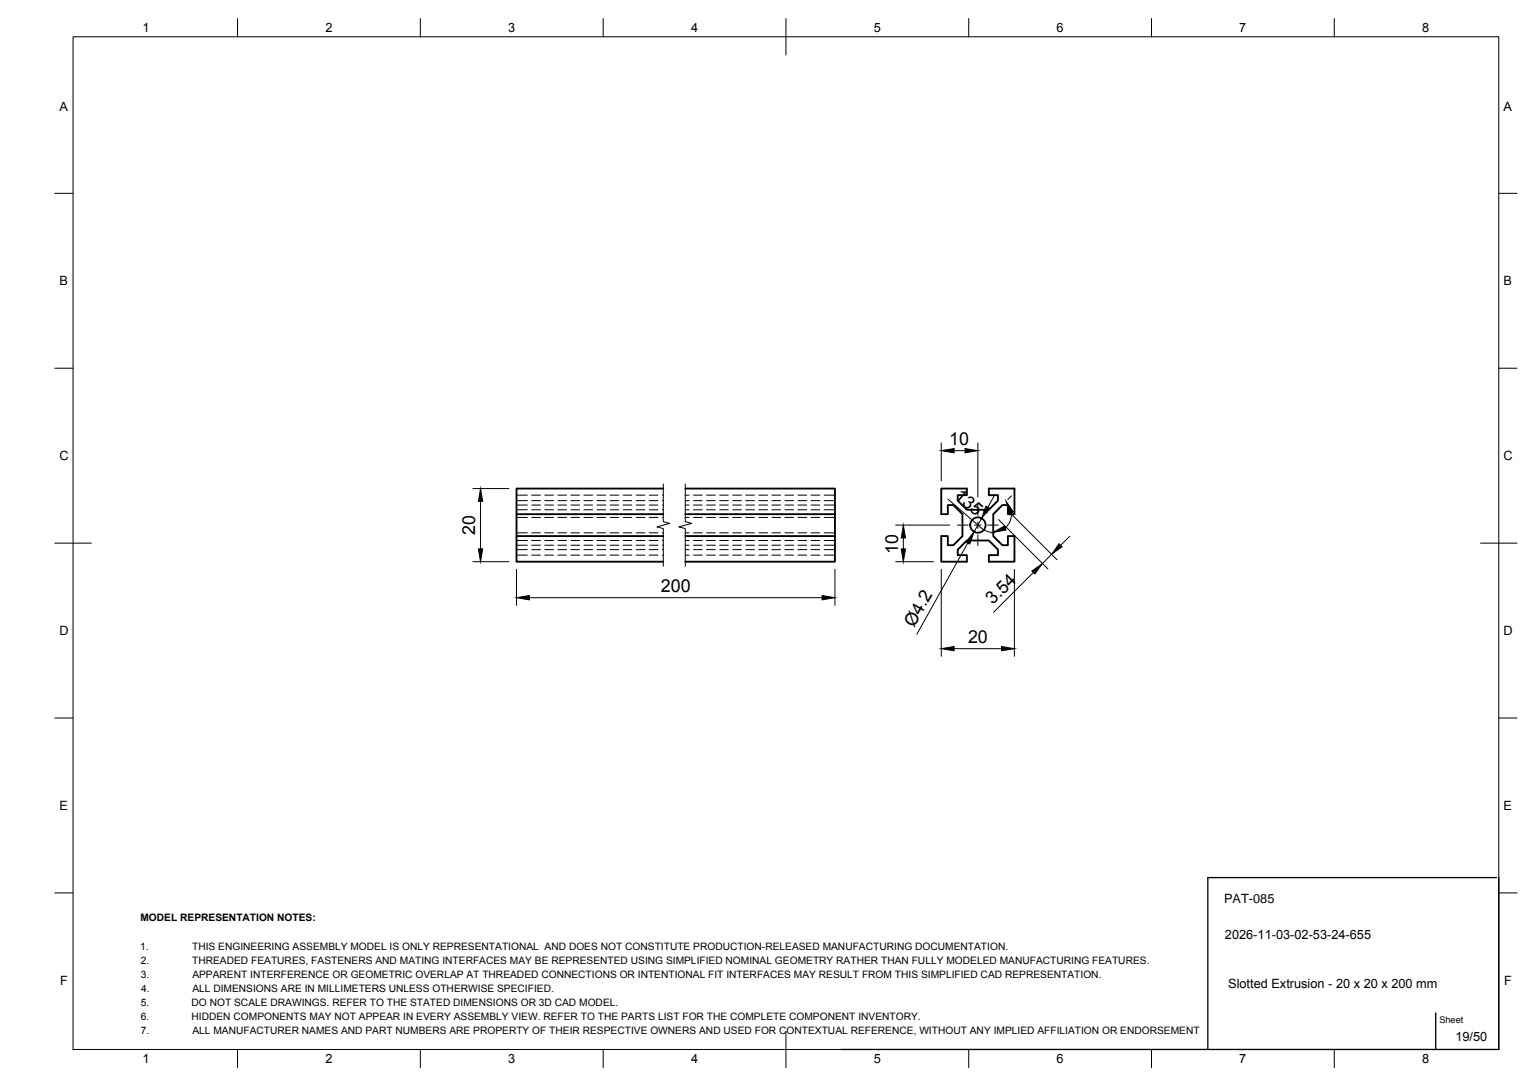
ISO-10303-21;
HEADER;
/* Generated by software containing ST-Developer
 * from STEP Tools, Inc. (www.steptools.com) 
 */

FILE_DESCRIPTION(
/* description */ ('Rack and pinion manual slide'),
/* implementation_level */ '2;1');

FILE_NAME(
/* name */ 'Slotted Extrusion - 20 x 20 x 200 mm.step',
/* time_stamp */ '2026-10-28T03:22:49-07:00',
/* author */ (''),
/* organization */ (''),
/* preprocessor_version */ 'ST-DEVELOPER v20.2',
/* originating_system */ 'Autodesk Translation Framework v15.17.0.0',
/* authorisation */ '');

FILE_SCHEMA (('AUTOMOTIVE_DESIGN { 1 0 10303 214 3 1 1 }'));
ENDSEC;

DATA;
#10=MECHANICAL_DESIGN_GEOMETRIC_PRESENTATION_REPRESENTATION('',(#746),#34851);
#654=SHAPE_REPRESENTATION_RELATIONSHIP('SRR','None',#35089,#700);
#700=ADVANCED_BREP_SHAPE_REPRESENTATION('',(#799),#34814);
#746=STYLED_ITEM('',(#35425),#799);
#799=MANIFOLD_SOLID_BREP('Body1',#13766);
#957=FACE_BOUND('',#2598,.T.);
#958=FACE_BOUND('',#2600,.T.);
#1128=PLANE('',#14628);
#1129=PLANE('',#14629);
#1130=PLANE('',#14630);
#1131=PLANE('',#14631);
#1132=PLANE('',#14632);
#1133=PLANE('',#14633);
#1134=PLANE('',#14634);
#1135=PLANE('',#14635);
#1136=PLANE('',#14636);
#1137=PLANE('',#14637);
#1138=PLANE('',#14638);
#1139=PLANE('',#14639);
#1140=PLANE('',#14640);
#1141=PLANE('',#14641);
#1142=PLANE('',#14642);
#1143=PLANE('',#14643);
#1144=PLANE('',#14644);
#1145=PLANE('',#14645);
#1146=PLANE('',#14646);
#1147=PLANE('',#14647);
#1148=PLANE('',#14648);
#1149=PLANE('',#14649);
#1150=PLANE('',#14650);
#1151=PLANE('',#14651);
#1152=PLANE('',#14652);
#1153=PLANE('',#14653);
#1154=PLANE('',#14654);
#1155=PLANE('',#14655);
#1156=PLANE('',#14656);
#1157=PLANE('',#14657);
#1158=PLANE('',#14658);
#1159=PLANE('',#14659);
#1160=PLANE('',#14660);
#1161=PLANE('',#14661);
#1162=PLANE('',#14662);
#1163=PLANE('',#14663);
#1164=PLANE('',#14667);
#1165=PLANE('',#14668);
#1166=PLANE('',#14669);
#1167=PLANE('',#14670);
#1168=PLANE('',#14671);
#1169=PLANE('',#14672);
#1170=PLANE('',#14673);
#1171=PLANE('',#14674);
#1172=PLANE('',#14675);
#1173=PLANE('',#14676);
#1689=FACE_OUTER_BOUND('',#2552,.T.);
#1690=FACE_OUTER_BOUND('',#2553,.T.);
#1691=FACE_OUTER_BOUND('',#2554,.T.);
#1692=FACE_OUTER_BOUND('',#2555,.T.);
#1693=FACE_OUTER_BOUND('',#2556,.T.);
#1694=FACE_OUTER_BOUND('',#2557,.T.);
#1695=FACE_OUTER_BOUND('',#2558,.T.);
#1696=FACE_OUTER_BOUND('',#2559,.T.);
#1697=FACE_OUTER_BOUND('',#2560,.T.);
#1698=FACE_OUTER_BOUND('',#2561,.T.);
#1699=FACE_OUTER_BOUND('',#2562,.T.);
#1700=FACE_OUTER_BOUND('',#2563,.T.);
#1701=FACE_OUTER_BOUND('',#2564,.T.);
#1702=FACE_OUTER_BOUND('',#2565,.T.);
#1703=FACE_OUTER_BOUND('',#2566,.T.);
#1704=FACE_OUTER_BOUND('',#2567,.T.);
#1705=FACE_OUTER_BOUND('',#2568,.T.);
#1706=FACE_OUTER_BOUND('',#2569,.T.);
#1707=FACE_OUTER_BOUND('',#2570,.T.);
#1708=FACE_OUTER_BOUND('',#2571,.T.);
#1709=FACE_OUTER_BOUND('',#2572,.T.);
#1710=FACE_OUTER_BOUND('',#2573,.T.);
#1711=FACE_OUTER_BOUND('',#2574,.T.);
#1712=FACE_OUTER_BOUND('',#2575,.T.);
#1713=FACE_OUTER_BOUND('',#2576,.T.);
#1714=FACE_OUTER_BOUND('',#2577,.T.);
#1715=FACE_OUTER_BOUND('',#2578,.T.);
#1716=FACE_OUTER_BOUND('',#2579,.T.);
#1717=FACE_OUTER_BOUND('',#2580,.T.);
#1718=FACE_OUTER_BOUND('',#2581,.T.);
#1719=FACE_OUTER_BOUND('',#2582,.T.);
#1720=FACE_OUTER_BOUND('',#2583,.T.);
#1721=FACE_OUTER_BOUND('',#2584,.T.);
#1722=FACE_OUTER_BOUND('',#2585,.T.);
#1723=FACE_OUTER_BOUND('',#2586,.T.);
#1724=FACE_OUTER_BOUND('',#2587,.T.);
#1725=FACE_OUTER_BOUND('',#2588,.T.);
#1726=FACE_OUTER_BOUND('',#2589,.T.);
#1727=FACE_OUTER_BOUND('',#2590,.T.);
#1728=FACE_OUTER_BOUND('',#2591,.T.);
#1729=FACE_OUTER_BOUND('',#2592,.T.);
#1730=FACE_OUTER_BOUND('',#2593,.T.);
#1731=FACE_OUTER_BOUND('',#2594,.T.);
#1732=FACE_OUTER_BOUND('',#2595,.T.);
#1733=FACE_OUTER_BOUND('',#2596,.T.);
#1734=FACE_OUTER_BOUND('',#2597,.T.);
#1735=FACE_OUTER_BOUND('',#2599,.T.);
#2552=EDGE_LOOP('',(#9942,#9943,#9944,#9945));
#2553=EDGE_LOOP('',(#9946,#9947,#9948,#9949));
#2554=EDGE_LOOP('',(#9950,#9951,#9952,#9953));
#2555=EDGE_LOOP('',(#9954,#9955,#9956,#9957));
#2556=EDGE_LOOP('',(#9958,#9959,#9960,#9961));
#2557=EDGE_LOOP('',(#9962,#9963,#9964,#9965));
#2558=EDGE_LOOP('',(#9966,#9967,#9968,#9969));
#2559=EDGE_LOOP('',(#9970,#9971,#9972,#9973));
#2560=EDGE_LOOP('',(#9974,#9975,#9976,#9977));
#2561=EDGE_LOOP('',(#9978,#9979,#9980,#9981));
#2562=EDGE_LOOP('',(#9982,#9983,#9984,#9985));
#2563=EDGE_LOOP('',(#9986,#9987,#9988,#9989));
#2564=EDGE_LOOP('',(#9990,#9991,#9992,#9993));
#2565=EDGE_LOOP('',(#9994,#9995,#9996,#9997));
#2566=EDGE_LOOP('',(#9998,#9999,#10000,#10001));
#2567=EDGE_LOOP('',(#10002,#10003,#10004,#10005));
#2568=EDGE_LOOP('',(#10006,#10007,#10008,#10009));
#2569=EDGE_LOOP('',(#10010,#10011,#10012,#10013));
#2570=EDGE_LOOP('',(#10014,#10015,#10016,#10017));
#2571=EDGE_LOOP('',(#10018,#10019,#10020,#10021));
#2572=EDGE_LOOP('',(#10022,#10023,#10024,#10025));
#2573=EDGE_LOOP('',(#10026,#10027,#10028,#10029));
#2574=EDGE_LOOP('',(#10030,#10031,#10032,#10033));
#2575=EDGE_LOOP('',(#10034,#10035,#10036,#10037));
#2576=EDGE_LOOP('',(#10038,#10039,#10040,#10041));
#2577=EDGE_LOOP('',(#10042,#10043,#10044,#10045));
#2578=EDGE_LOOP('',(#10046,#10047,#10048,#10049));
#2579=EDGE_LOOP('',(#10050,#10051,#10052,#10053));
#2580=EDGE_LOOP('',(#10054,#10055,#10056,#10057));
#2581=EDGE_LOOP('',(#10058,#10059,#10060,#10061));
#2582=EDGE_LOOP('',(#10062,#10063,#10064,#10065));
#2583=EDGE_LOOP('',(#10066,#10067,#10068,#10069));
#2584=EDGE_LOOP('',(#10070,#10071,#10072,#10073));
#2585=EDGE_LOOP('',(#10074,#10075,#10076,#10077));
#2586=EDGE_LOOP('',(#10078,#10079,#10080,#10081));
#2587=EDGE_LOOP('',(#10082,#10083,#10084,#10085));
#2588=EDGE_LOOP('',(#10086,#10087,#10088,#10089));
#2589=EDGE_LOOP('',(#10090,#10091,#10092,#10093));
#2590=EDGE_LOOP('',(#10094,#10095,#10096,#10097));
#2591=EDGE_LOOP('',(#10098,#10099,#10100,#10101));
#2592=EDGE_LOOP('',(#10102,#10103,#10104,#10105));
#2593=EDGE_LOOP('',(#10106,#10107,#10108,#10109));
#2594=EDGE_LOOP('',(#10110,#10111,#10112,#10113));
#2595=EDGE_LOOP('',(#10114,#10115,#10116,#10117));
#2596=EDGE_LOOP('',(#10118,#10119,#10120,#10121));
#2597=EDGE_LOOP('',(#10122,#10123,#10124,#10125,#10126,#10127,#10128,#10129,
#10130,#10131,#10132,#10133,#10134,#10135,#10136,#10137,#10138,#10139,#10140,
#10141,#10142,#10143,#10144,#10145,#10146,#10147,#10148,#10149,#10150,#10151,
#10152,#10153,#10154,#10155,#10156,#10157,#10158,#10159,#10160,#10161,#10162,
#10163,#10164,#10165));
#2598=EDGE_LOOP('',(#10166));
#2599=EDGE_LOOP('',(#10167,#10168,#10169,#10170,#10171,#10172,#10173,#10174,
#10175,#10176,#10177,#10178,#10179,#10180,#10181,#10182,#10183,#10184,#10185,
#10186,#10187,#10188,#10189,#10190,#10191,#10192,#10193,#10194,#10195,#10196,
#10197,#10198,#10199,#10200,#10201,#10202,#10203,#10204,#10205,#10206,#10207,
#10208,#10209,#10210));
#2600=EDGE_LOOP('',(#10211));
#3438=LINE('',#20221,#4729);
#3439=LINE('',#20223,#4730);
#3440=LINE('',#20225,#4731);
#3441=LINE('',#20226,#4732);
#3442=LINE('',#20229,#4733);
#3443=LINE('',#20231,#4734);
#3444=LINE('',#20232,#4735);
#3445=LINE('',#20235,#4736);
#3446=LINE('',#20237,#4737);
#3447=LINE('',#20238,#4738);
#3448=LINE('',#20241,#4739);
#3449=LINE('',#20243,#4740);
#3450=LINE('',#20244,#4741);
#3451=LINE('',#20247,#4742);
#3452=LINE('',#20249,#4743);
#3453=LINE('',#20250,#4744);
#3454=LINE('',#20253,#4745);
#3455=LINE('',#20255,#4746);
#3456=LINE('',#20256,#4747);
#3457=LINE('',#20259,#4748);
#3458=LINE('',#20261,#4749);
#3459=LINE('',#20262,#4750);
#3460=LINE('',#20265,#4751);
#3461=LINE('',#20267,#4752);
#3462=LINE('',#20268,#4753);
#3463=LINE('',#20271,#4754);
#3464=LINE('',#20273,#4755);
#3465=LINE('',#20274,#4756);
#3466=LINE('',#20278,#4757);
#3467=LINE('',#20280,#4758);
#3468=LINE('',#20282,#4759);
#3469=LINE('',#20283,#4760);
#3470=LINE('',#20286,#4761);
#3471=LINE('',#20288,#4762);
#3472=LINE('',#20289,#4763);
#3473=LINE('',#20292,#4764);
#3474=LINE('',#20294,#4765);
#3475=LINE('',#20295,#4766);
#3476=LINE('',#20298,#4767);
#3477=LINE('',#20300,#4768);
#3478=LINE('',#20301,#4769);
#3479=LINE('',#20304,#4770);
#3480=LINE('',#20306,#4771);
#3481=LINE('',#20307,#4772);
#3482=LINE('',#20310,#4773);
#3483=LINE('',#20312,#4774);
#3484=LINE('',#20313,#4775);
#3485=LINE('',#20316,#4776);
#3486=LINE('',#20318,#4777);
#3487=LINE('',#20319,#4778);
#3488=LINE('',#20322,#4779);
#3489=LINE('',#20324,#4780);
#3490=LINE('',#20325,#4781);
#3491=LINE('',#20328,#4782);
#3492=LINE('',#20330,#4783);
#3493=LINE('',#20331,#4784);
#3494=LINE('',#20335,#4785);
#3495=LINE('',#20337,#4786);
#3496=LINE('',#20339,#4787);
#3497=LINE('',#20340,#4788);
#3498=LINE('',#20343,#4789);
#3499=LINE('',#20345,#4790);
#3500=LINE('',#20346,#4791);
#3501=LINE('',#20349,#4792);
#3502=LINE('',#20351,#4793);
#3503=LINE('',#20352,#4794);
#3504=LINE('',#20355,#4795);
#3505=LINE('',#20357,#4796);
#3506=LINE('',#20358,#4797);
#3507=LINE('',#20361,#4798);
#3508=LINE('',#20363,#4799);
#3509=LINE('',#20364,#4800);
#3510=LINE('',#20367,#4801);
#3511=LINE('',#20369,#4802);
#3512=LINE('',#20370,#4803);
#3513=LINE('',#20373,#4804);
#3514=LINE('',#20375,#4805);
#3515=LINE('',#20376,#4806);
#3516=LINE('',#20379,#4807);
#3517=LINE('',#20381,#4808);
#3518=LINE('',#20382,#4809);
#3519=LINE('',#20385,#4810);
#3520=LINE('',#20387,#4811);
#3521=LINE('',#20388,#4812);
#3522=LINE('',#20392,#4813);
#3523=LINE('',#20394,#4814);
#3524=LINE('',#20396,#4815);
#3525=LINE('',#20397,#4816);
#3526=LINE('',#20400,#4817);
#3527=LINE('',#20402,#4818);
#3528=LINE('',#20403,#4819);
#3529=LINE('',#20406,#4820);
#3530=LINE('',#20408,#4821);
#3531=LINE('',#20409,#4822);
#3532=LINE('',#20412,#4823);
#3533=LINE('',#20414,#4824);
#3534=LINE('',#20415,#4825);
#3535=LINE('',#20418,#4826);
#3536=LINE('',#20420,#4827);
#3537=LINE('',#20421,#4828);
#3538=LINE('',#20424,#4829);
#3539=LINE('',#20426,#4830);
#3540=LINE('',#20427,#4831);
#3541=LINE('',#20430,#4832);
#3542=LINE('',#20432,#4833);
#3543=LINE('',#20433,#4834);
#3544=LINE('',#20436,#4835);
#3545=LINE('',#20438,#4836);
#3546=LINE('',#20439,#4837);
#3547=LINE('',#20442,#4838);
#3548=LINE('',#20444,#4839);
#3549=LINE('',#20445,#4840);
#3550=LINE('',#20450,#4841);
#3551=LINE('',#20454,#4842);
#3552=LINE('',#20456,#4843);
#3553=LINE('',#20457,#4844);
#3554=LINE('',#20460,#4845);
#3555=LINE('',#20462,#4846);
#3556=LINE('',#20463,#4847);
#3557=LINE('',#20465,#4848);
#3558=LINE('',#20466,#4849);
#3559=LINE('',#20469,#4850);
#3560=LINE('',#20471,#4851);
#3561=LINE('',#20472,#4852);
#3562=LINE('',#20474,#4853);
#3563=LINE('',#20475,#4854);
#3564=LINE('',#20478,#4855);
#3565=LINE('',#20480,#4856);
#3566=LINE('',#20481,#4857);
#3567=LINE('',#20483,#4858);
#3568=LINE('',#20484,#4859);
#3569=LINE('',#20486,#4860);
#3570=LINE('',#20487,#4861);
#4729=VECTOR('',#16438,1.);
#4730=VECTOR('',#16439,1.);
#4731=VECTOR('',#16440,1.);
#4732=VECTOR('',#16441,1.);
#4733=VECTOR('',#16444,1.);
#4734=VECTOR('',#16445,1.);
#4735=VECTOR('',#16446,1.);
#4736=VECTOR('',#16449,1.);
#4737=VECTOR('',#16450,1.);
#4738=VECTOR('',#16451,1.);
#4739=VECTOR('',#16454,1.);
#4740=VECTOR('',#16455,1.);
#4741=VECTOR('',#16456,1.);
#4742=VECTOR('',#16459,1.);
#4743=VECTOR('',#16460,1.);
#4744=VECTOR('',#16461,1.);
#4745=VECTOR('',#16464,1.);
#4746=VECTOR('',#16465,1.);
#4747=VECTOR('',#16466,1.);
#4748=VECTOR('',#16469,1.);
#4749=VECTOR('',#16470,1.);
#4750=VECTOR('',#16471,1.);
#4751=VECTOR('',#16474,1.);
#4752=VECTOR('',#16475,1.);
#4753=VECTOR('',#16476,1.);
#4754=VECTOR('',#16479,1.);
#4755=VECTOR('',#16480,1.);
#4756=VECTOR('',#16481,1.);
#4757=VECTOR('',#16484,1.);
#4758=VECTOR('',#16485,1.);
#4759=VECTOR('',#16486,1.);
#4760=VECTOR('',#16487,1.);
#4761=VECTOR('',#16490,1.);
#4762=VECTOR('',#16491,1.);
#4763=VECTOR('',#16492,1.);
#4764=VECTOR('',#16495,1.);
#4765=VECTOR('',#16496,1.);
#4766=VECTOR('',#16497,1.);
#4767=VECTOR('',#16500,1.);
#4768=VECTOR('',#16501,1.);
#4769=VECTOR('',#16502,1.);
#4770=VECTOR('',#16505,1.);
#4771=VECTOR('',#16506,1.);
#4772=VECTOR('',#16507,1.);
#4773=VECTOR('',#16510,1.);
#4774=VECTOR('',#16511,1.);
#4775=VECTOR('',#16512,1.);
#4776=VECTOR('',#16515,1.);
#4777=VECTOR('',#16516,1.);
#4778=VECTOR('',#16517,1.);
#4779=VECTOR('',#16520,1.);
#4780=VECTOR('',#16521,1.);
#4781=VECTOR('',#16522,1.);
#4782=VECTOR('',#16525,1.);
#4783=VECTOR('',#16526,1.);
#4784=VECTOR('',#16527,1.);
#4785=VECTOR('',#16530,1.);
#4786=VECTOR('',#16531,1.);
#4787=VECTOR('',#16532,1.);
#4788=VECTOR('',#16533,1.);
#4789=VECTOR('',#16536,1.);
#4790=VECTOR('',#16537,1.);
#4791=VECTOR('',#16538,1.);
#4792=VECTOR('',#16541,1.);
#4793=VECTOR('',#16542,1.);
#4794=VECTOR('',#16543,1.);
#4795=VECTOR('',#16546,1.);
#4796=VECTOR('',#16547,1.);
#4797=VECTOR('',#16548,1.);
#4798=VECTOR('',#16551,1.);
#4799=VECTOR('',#16552,1.);
#4800=VECTOR('',#16553,1.);
#4801=VECTOR('',#16556,1.);
#4802=VECTOR('',#16557,1.);
#4803=VECTOR('',#16558,1.);
#4804=VECTOR('',#16561,1.);
#4805=VECTOR('',#16562,1.);
#4806=VECTOR('',#16563,1.);
#4807=VECTOR('',#16566,1.);
#4808=VECTOR('',#16567,1.);
#4809=VECTOR('',#16568,1.);
#4810=VECTOR('',#16571,1.);
#4811=VECTOR('',#16572,1.);
#4812=VECTOR('',#16573,1.);
#4813=VECTOR('',#16576,1.);
#4814=VECTOR('',#16577,1.);
#4815=VECTOR('',#16578,1.);
#4816=VECTOR('',#16579,1.);
#4817=VECTOR('',#16582,1.);
#4818=VECTOR('',#16583,1.);
#4819=VECTOR('',#16584,1.);
#4820=VECTOR('',#16587,1.);
#4821=VECTOR('',#16588,1.);
#4822=VECTOR('',#16589,1.);
#4823=VECTOR('',#16592,1.);
#4824=VECTOR('',#16593,1.);
#4825=VECTOR('',#16594,1.);
#4826=VECTOR('',#16597,1.);
#4827=VECTOR('',#16598,1.);
#4828=VECTOR('',#16599,1.);
#4829=VECTOR('',#16602,1.);
#4830=VECTOR('',#16603,1.);
#4831=VECTOR('',#16604,1.);
#4832=VECTOR('',#16607,1.);
#4833=VECTOR('',#16608,1.);
#4834=VECTOR('',#16609,1.);
#4835=VECTOR('',#16612,1.);
#4836=VECTOR('',#16613,1.);
#4837=VECTOR('',#16614,1.);
#4838=VECTOR('',#16617,1.);
#4839=VECTOR('',#16618,1.);
#4840=VECTOR('',#16619,1.);
#4841=VECTOR('',#16624,0.21);
#4842=VECTOR('',#16629,1.);
#4843=VECTOR('',#16630,1.);
#4844=VECTOR('',#16631,1.);
#4845=VECTOR('',#16634,1.);
#4846=VECTOR('',#16635,1.);
#4847=VECTOR('',#16636,1.);
#4848=VECTOR('',#16639,1.);
#4849=VECTOR('',#16640,1.);
#4850=VECTOR('',#16643,1.);
#4851=VECTOR('',#16644,1.);
#4852=VECTOR('',#16645,1.);
#4853=VECTOR('',#16648,1.);
#4854=VECTOR('',#16649,1.);
#4855=VECTOR('',#16652,1.);
#4856=VECTOR('',#16653,1.);
#4857=VECTOR('',#16654,1.);
#4858=VECTOR('',#16657,1.);
#4859=VECTOR('',#16658,1.);
#4860=VECTOR('',#16661,1.);
#4861=VECTOR('',#16662,1.);
#5946=CIRCLE('',#14665,0.21);
#5947=CIRCLE('',#14666,0.21);
#6460=VERTEX_POINT('',#20219);
#6461=VERTEX_POINT('',#20220);
#6462=VERTEX_POINT('',#20222);
#6463=VERTEX_POINT('',#20224);
#6464=VERTEX_POINT('',#20228);
#6465=VERTEX_POINT('',#20230);
#6466=VERTEX_POINT('',#20234);
#6467=VERTEX_POINT('',#20236);
#6468=VERTEX_POINT('',#20240);
#6469=VERTEX_POINT('',#20242);
#6470=VERTEX_POINT('',#20246);
#6471=VERTEX_POINT('',#20248);
#6472=VERTEX_POINT('',#20252);
#6473=VERTEX_POINT('',#20254);
#6474=VERTEX_POINT('',#20258);
#6475=VERTEX_POINT('',#20260);
#6476=VERTEX_POINT('',#20264);
#6477=VERTEX_POINT('',#20266);
#6478=VERTEX_POINT('',#20270);
#6479=VERTEX_POINT('',#20272);
#6480=VERTEX_POINT('',#20276);
#6481=VERTEX_POINT('',#20277);
#6482=VERTEX_POINT('',#20279);
#6483=VERTEX_POINT('',#20281);
#6484=VERTEX_POINT('',#20285);
#6485=VERTEX_POINT('',#20287);
#6486=VERTEX_POINT('',#20291);
#6487=VERTEX_POINT('',#20293);
#6488=VERTEX_POINT('',#20297);
#6489=VERTEX_POINT('',#20299);
#6490=VERTEX_POINT('',#20303);
#6491=VERTEX_POINT('',#20305);
#6492=VERTEX_POINT('',#20309);
#6493=VERTEX_POINT('',#20311);
#6494=VERTEX_POINT('',#20315);
#6495=VERTEX_POINT('',#20317);
#6496=VERTEX_POINT('',#20321);
#6497=VERTEX_POINT('',#20323);
#6498=VERTEX_POINT('',#20327);
#6499=VERTEX_POINT('',#20329);
#6500=VERTEX_POINT('',#20333);
#6501=VERTEX_POINT('',#20334);
#6502=VERTEX_POINT('',#20336);
#6503=VERTEX_POINT('',#20338);
#6504=VERTEX_POINT('',#20342);
#6505=VERTEX_POINT('',#20344);
#6506=VERTEX_POINT('',#20348);
#6507=VERTEX_POINT('',#20350);
#6508=VERTEX_POINT('',#20354);
#6509=VERTEX_POINT('',#20356);
#6510=VERTEX_POINT('',#20360);
#6511=VERTEX_POINT('',#20362);
#6512=VERTEX_POINT('',#20366);
#6513=VERTEX_POINT('',#20368);
#6514=VERTEX_POINT('',#20372);
#6515=VERTEX_POINT('',#20374);
#6516=VERTEX_POINT('',#20378);
#6517=VERTEX_POINT('',#20380);
#6518=VERTEX_POINT('',#20384);
#6519=VERTEX_POINT('',#20386);
#6520=VERTEX_POINT('',#20390);
#6521=VERTEX_POINT('',#20391);
#6522=VERTEX_POINT('',#20393);
#6523=VERTEX_POINT('',#20395);
#6524=VERTEX_POINT('',#20399);
#6525=VERTEX_POINT('',#20401);
#6526=VERTEX_POINT('',#20405);
#6527=VERTEX_POINT('',#20407);
#6528=VERTEX_POINT('',#20411);
#6529=VERTEX_POINT('',#20413);
#6530=VERTEX_POINT('',#20417);
#6531=VERTEX_POINT('',#20419);
#6532=VERTEX_POINT('',#20423);
#6533=VERTEX_POINT('',#20425);
#6534=VERTEX_POINT('',#20429);
#6535=VERTEX_POINT('',#20431);
#6536=VERTEX_POINT('',#20435);
#6537=VERTEX_POINT('',#20437);
#6538=VERTEX_POINT('',#20441);
#6539=VERTEX_POINT('',#20443);
#6540=VERTEX_POINT('',#20447);
#6541=VERTEX_POINT('',#20449);
#6542=VERTEX_POINT('',#20453);
#6543=VERTEX_POINT('',#20455);
#6544=VERTEX_POINT('',#20459);
#6545=VERTEX_POINT('',#20461);
#6546=VERTEX_POINT('',#20468);
#6547=VERTEX_POINT('',#20470);
#6548=VERTEX_POINT('',#20477);
#6549=VERTEX_POINT('',#20479);
#7783=EDGE_CURVE('',#6460,#6461,#3438,.T.);
#7784=EDGE_CURVE('',#6460,#6462,#3439,.T.);
#7785=EDGE_CURVE('',#6463,#6462,#3440,.T.);
#7786=EDGE_CURVE('',#6461,#6463,#3441,.T.);
#7787=EDGE_CURVE('',#6464,#6460,#3442,.T.);
#7788=EDGE_CURVE('',#6464,#6465,#3443,.T.);
#7789=EDGE_CURVE('',#6462,#6465,#3444,.T.);
#7790=EDGE_CURVE('',#6466,#6464,#3445,.T.);
#7791=EDGE_CURVE('',#6466,#6467,#3446,.T.);
#7792=EDGE_CURVE('',#6465,#6467,#3447,.T.);
#7793=EDGE_CURVE('',#6468,#6466,#3448,.T.);
#7794=EDGE_CURVE('',#6468,#6469,#3449,.T.);
#7795=EDGE_CURVE('',#6467,#6469,#3450,.T.);
#7796=EDGE_CURVE('',#6470,#6468,#3451,.T.);
#7797=EDGE_CURVE('',#6470,#6471,#3452,.T.);
#7798=EDGE_CURVE('',#6469,#6471,#3453,.T.);
#7799=EDGE_CURVE('',#6472,#6470,#3454,.T.);
#7800=EDGE_CURVE('',#6472,#6473,#3455,.T.);
#7801=EDGE_CURVE('',#6471,#6473,#3456,.T.);
#7802=EDGE_CURVE('',#6474,#6472,#3457,.T.);
#7803=EDGE_CURVE('',#6474,#6475,#3458,.T.);
#7804=EDGE_CURVE('',#6473,#6475,#3459,.T.);
#7805=EDGE_CURVE('',#6476,#6474,#3460,.T.);
#7806=EDGE_CURVE('',#6476,#6477,#3461,.T.);
#7807=EDGE_CURVE('',#6475,#6477,#3462,.T.);
#7808=EDGE_CURVE('',#6478,#6476,#3463,.T.);
#7809=EDGE_CURVE('',#6479,#6478,#3464,.T.);
#7810=EDGE_CURVE('',#6477,#6479,#3465,.T.);
#7811=EDGE_CURVE('',#6480,#6481,#3466,.T.);
#7812=EDGE_CURVE('',#6480,#6482,#3467,.T.);
#7813=EDGE_CURVE('',#6483,#6482,#3468,.T.);
#7814=EDGE_CURVE('',#6481,#6483,#3469,.T.);
#7815=EDGE_CURVE('',#6484,#6480,#3470,.T.);
#7816=EDGE_CURVE('',#6484,#6485,#3471,.T.);
#7817=EDGE_CURVE('',#6482,#6485,#3472,.T.);
#7818=EDGE_CURVE('',#6486,#6484,#3473,.T.);
#7819=EDGE_CURVE('',#6486,#6487,#3474,.T.);
#7820=EDGE_CURVE('',#6485,#6487,#3475,.T.);
#7821=EDGE_CURVE('',#6488,#6486,#3476,.T.);
#7822=EDGE_CURVE('',#6488,#6489,#3477,.T.);
#7823=EDGE_CURVE('',#6487,#6489,#3478,.T.);
#7824=EDGE_CURVE('',#6490,#6488,#3479,.T.);
#7825=EDGE_CURVE('',#6490,#6491,#3480,.T.);
#7826=EDGE_CURVE('',#6489,#6491,#3481,.T.);
#7827=EDGE_CURVE('',#6492,#6490,#3482,.T.);
#7828=EDGE_CURVE('',#6492,#6493,#3483,.T.);
#7829=EDGE_CURVE('',#6491,#6493,#3484,.T.);
#7830=EDGE_CURVE('',#6494,#6492,#3485,.T.);
#7831=EDGE_CURVE('',#6494,#6495,#3486,.T.);
#7832=EDGE_CURVE('',#6493,#6495,#3487,.T.);
#7833=EDGE_CURVE('',#6496,#6494,#3488,.T.);
#7834=EDGE_CURVE('',#6496,#6497,#3489,.T.);
#7835=EDGE_CURVE('',#6495,#6497,#3490,.T.);
#7836=EDGE_CURVE('',#6498,#6496,#3491,.T.);
#7837=EDGE_CURVE('',#6499,#6498,#3492,.T.);
#7838=EDGE_CURVE('',#6497,#6499,#3493,.T.);
#7839=EDGE_CURVE('',#6500,#6501,#3494,.T.);
#7840=EDGE_CURVE('',#6500,#6502,#3495,.T.);
#7841=EDGE_CURVE('',#6503,#6502,#3496,.T.);
#7842=EDGE_CURVE('',#6501,#6503,#3497,.T.);
#7843=EDGE_CURVE('',#6504,#6500,#3498,.T.);
#7844=EDGE_CURVE('',#6504,#6505,#3499,.T.);
#7845=EDGE_CURVE('',#6502,#6505,#3500,.T.);
#7846=EDGE_CURVE('',#6506,#6504,#3501,.T.);
#7847=EDGE_CURVE('',#6506,#6507,#3502,.T.);
#7848=EDGE_CURVE('',#6505,#6507,#3503,.T.);
#7849=EDGE_CURVE('',#6508,#6506,#3504,.T.);
#7850=EDGE_CURVE('',#6508,#6509,#3505,.T.);
#7851=EDGE_CURVE('',#6507,#6509,#3506,.T.);
#7852=EDGE_CURVE('',#6510,#6508,#3507,.T.);
#7853=EDGE_CURVE('',#6510,#6511,#3508,.T.);
#7854=EDGE_CURVE('',#6509,#6511,#3509,.T.);
#7855=EDGE_CURVE('',#6512,#6510,#3510,.T.);
#7856=EDGE_CURVE('',#6512,#6513,#3511,.T.);
#7857=EDGE_CURVE('',#6511,#6513,#3512,.T.);
#7858=EDGE_CURVE('',#6514,#6512,#3513,.T.);
#7859=EDGE_CURVE('',#6514,#6515,#3514,.T.);
#7860=EDGE_CURVE('',#6513,#6515,#3515,.T.);
#7861=EDGE_CURVE('',#6516,#6514,#3516,.T.);
#7862=EDGE_CURVE('',#6516,#6517,#3517,.T.);
#7863=EDGE_CURVE('',#6515,#6517,#3518,.T.);
#7864=EDGE_CURVE('',#6518,#6516,#3519,.T.);
#7865=EDGE_CURVE('',#6519,#6518,#3520,.T.);
#7866=EDGE_CURVE('',#6517,#6519,#3521,.T.);
#7867=EDGE_CURVE('',#6520,#6521,#3522,.T.);
#7868=EDGE_CURVE('',#6520,#6522,#3523,.T.);
#7869=EDGE_CURVE('',#6523,#6522,#3524,.T.);
#7870=EDGE_CURVE('',#6521,#6523,#3525,.T.);
#7871=EDGE_CURVE('',#6524,#6520,#3526,.T.);
#7872=EDGE_CURVE('',#6524,#6525,#3527,.T.);
#7873=EDGE_CURVE('',#6522,#6525,#3528,.T.);
#7874=EDGE_CURVE('',#6526,#6524,#3529,.T.);
#7875=EDGE_CURVE('',#6526,#6527,#3530,.T.);
#7876=EDGE_CURVE('',#6525,#6527,#3531,.T.);
#7877=EDGE_CURVE('',#6528,#6526,#3532,.T.);
#7878=EDGE_CURVE('',#6528,#6529,#3533,.T.);
#7879=EDGE_CURVE('',#6527,#6529,#3534,.T.);
#7880=EDGE_CURVE('',#6530,#6528,#3535,.T.);
#7881=EDGE_CURVE('',#6530,#6531,#3536,.T.);
#7882=EDGE_CURVE('',#6529,#6531,#3537,.T.);
#7883=EDGE_CURVE('',#6532,#6530,#3538,.T.);
#7884=EDGE_CURVE('',#6532,#6533,#3539,.T.);
#7885=EDGE_CURVE('',#6531,#6533,#3540,.T.);
#7886=EDGE_CURVE('',#6534,#6532,#3541,.T.);
#7887=EDGE_CURVE('',#6534,#6535,#3542,.T.);
#7888=EDGE_CURVE('',#6533,#6535,#3543,.T.);
#7889=EDGE_CURVE('',#6536,#6534,#3544,.T.);
#7890=EDGE_CURVE('',#6536,#6537,#3545,.T.);
#7891=EDGE_CURVE('',#6535,#6537,#3546,.T.);
#7892=EDGE_CURVE('',#6538,#6536,#3547,.T.);
#7893=EDGE_CURVE('',#6539,#6538,#3548,.T.);
#7894=EDGE_CURVE('',#6537,#6539,#3549,.T.);
#7895=EDGE_CURVE('',#6540,#6540,#5946,.T.);
#7896=EDGE_CURVE('',#6540,#6541,#3550,.T.);
#7897=EDGE_CURVE('',#6541,#6541,#5947,.T.);
#7898=EDGE_CURVE('',#6478,#6542,#3551,.T.);
#7899=EDGE_CURVE('',#6542,#6543,#3552,.T.);
#7900=EDGE_CURVE('',#6479,#6543,#3553,.T.);
#7901=EDGE_CURVE('',#6544,#6463,#3554,.T.);
#7902=EDGE_CURVE('',#6545,#6544,#3555,.T.);
#7903=EDGE_CURVE('',#6545,#6461,#3556,.T.);
#7904=EDGE_CURVE('',#6498,#6545,#3557,.T.);
#7905=EDGE_CURVE('',#6499,#6544,#3558,.T.);
#7906=EDGE_CURVE('',#6546,#6483,#3559,.T.);
#7907=EDGE_CURVE('',#6547,#6546,#3560,.T.);
#7908=EDGE_CURVE('',#6547,#6481,#3561,.T.);
#7909=EDGE_CURVE('',#6518,#6547,#3562,.T.);
#7910=EDGE_CURVE('',#6519,#6546,#3563,.T.);
#7911=EDGE_CURVE('',#6548,#6503,#3564,.T.);
#7912=EDGE_CURVE('',#6549,#6548,#3565,.T.);
#7913=EDGE_CURVE('',#6549,#6501,#3566,.T.);
#7914=EDGE_CURVE('',#6538,#6549,#3567,.T.);
#7915=EDGE_CURVE('',#6539,#6548,#3568,.T.);
#7916=EDGE_CURVE('',#6543,#6523,#3569,.T.);
#7917=EDGE_CURVE('',#6542,#6521,#3570,.T.);
#9942=ORIENTED_EDGE('',*,*,#7783,.F.);
#9943=ORIENTED_EDGE('',*,*,#7784,.T.);
#9944=ORIENTED_EDGE('',*,*,#7785,.F.);
#9945=ORIENTED_EDGE('',*,*,#7786,.F.);
#9946=ORIENTED_EDGE('',*,*,#7787,.F.);
#9947=ORIENTED_EDGE('',*,*,#7788,.T.);
#9948=ORIENTED_EDGE('',*,*,#7789,.F.);
#9949=ORIENTED_EDGE('',*,*,#7784,.F.);
#9950=ORIENTED_EDGE('',*,*,#7790,.F.);
#9951=ORIENTED_EDGE('',*,*,#7791,.T.);
#9952=ORIENTED_EDGE('',*,*,#7792,.F.);
#9953=ORIENTED_EDGE('',*,*,#7788,.F.);
#9954=ORIENTED_EDGE('',*,*,#7793,.F.);
#9955=ORIENTED_EDGE('',*,*,#7794,.T.);
#9956=ORIENTED_EDGE('',*,*,#7795,.F.);
#9957=ORIENTED_EDGE('',*,*,#7791,.F.);
#9958=ORIENTED_EDGE('',*,*,#7796,.F.);
#9959=ORIENTED_EDGE('',*,*,#7797,.T.);
#9960=ORIENTED_EDGE('',*,*,#7798,.F.);
#9961=ORIENTED_EDGE('',*,*,#7794,.F.);
#9962=ORIENTED_EDGE('',*,*,#7799,.F.);
#9963=ORIENTED_EDGE('',*,*,#7800,.T.);
#9964=ORIENTED_EDGE('',*,*,#7801,.F.);
#9965=ORIENTED_EDGE('',*,*,#7797,.F.);
#9966=ORIENTED_EDGE('',*,*,#7802,.F.);
#9967=ORIENTED_EDGE('',*,*,#7803,.T.);
#9968=ORIENTED_EDGE('',*,*,#7804,.F.);
#9969=ORIENTED_EDGE('',*,*,#7800,.F.);
#9970=ORIENTED_EDGE('',*,*,#7805,.F.);
#9971=ORIENTED_EDGE('',*,*,#7806,.T.);
#9972=ORIENTED_EDGE('',*,*,#7807,.F.);
#9973=ORIENTED_EDGE('',*,*,#7803,.F.);
#9974=ORIENTED_EDGE('',*,*,#7808,.F.);
#9975=ORIENTED_EDGE('',*,*,#7809,.F.);
#9976=ORIENTED_EDGE('',*,*,#7810,.F.);
#9977=ORIENTED_EDGE('',*,*,#7806,.F.);
#9978=ORIENTED_EDGE('',*,*,#7811,.F.);
#9979=ORIENTED_EDGE('',*,*,#7812,.T.);
#9980=ORIENTED_EDGE('',*,*,#7813,.F.);
#9981=ORIENTED_EDGE('',*,*,#7814,.F.);
#9982=ORIENTED_EDGE('',*,*,#7815,.F.);
#9983=ORIENTED_EDGE('',*,*,#7816,.T.);
#9984=ORIENTED_EDGE('',*,*,#7817,.F.);
#9985=ORIENTED_EDGE('',*,*,#7812,.F.);
#9986=ORIENTED_EDGE('',*,*,#7818,.F.);
#9987=ORIENTED_EDGE('',*,*,#7819,.T.);
#9988=ORIENTED_EDGE('',*,*,#7820,.F.);
#9989=ORIENTED_EDGE('',*,*,#7816,.F.);
#9990=ORIENTED_EDGE('',*,*,#7821,.F.);
#9991=ORIENTED_EDGE('',*,*,#7822,.T.);
#9992=ORIENTED_EDGE('',*,*,#7823,.F.);
#9993=ORIENTED_EDGE('',*,*,#7819,.F.);
#9994=ORIENTED_EDGE('',*,*,#7824,.F.);
#9995=ORIENTED_EDGE('',*,*,#7825,.T.);
#9996=ORIENTED_EDGE('',*,*,#7826,.F.);
#9997=ORIENTED_EDGE('',*,*,#7822,.F.);
#9998=ORIENTED_EDGE('',*,*,#7827,.F.);
#9999=ORIENTED_EDGE('',*,*,#7828,.T.);
#10000=ORIENTED_EDGE('',*,*,#7829,.F.);
#10001=ORIENTED_EDGE('',*,*,#7825,.F.);
#10002=ORIENTED_EDGE('',*,*,#7830,.F.);
#10003=ORIENTED_EDGE('',*,*,#7831,.T.);
#10004=ORIENTED_EDGE('',*,*,#7832,.F.);
#10005=ORIENTED_EDGE('',*,*,#7828,.F.);
#10006=ORIENTED_EDGE('',*,*,#7833,.F.);
#10007=ORIENTED_EDGE('',*,*,#7834,.T.);
#10008=ORIENTED_EDGE('',*,*,#7835,.F.);
#10009=ORIENTED_EDGE('',*,*,#7831,.F.);
#10010=ORIENTED_EDGE('',*,*,#7836,.F.);
#10011=ORIENTED_EDGE('',*,*,#7837,.F.);
#10012=ORIENTED_EDGE('',*,*,#7838,.F.);
#10013=ORIENTED_EDGE('',*,*,#7834,.F.);
#10014=ORIENTED_EDGE('',*,*,#7839,.F.);
#10015=ORIENTED_EDGE('',*,*,#7840,.T.);
#10016=ORIENTED_EDGE('',*,*,#7841,.F.);
#10017=ORIENTED_EDGE('',*,*,#7842,.F.);
#10018=ORIENTED_EDGE('',*,*,#7843,.F.);
#10019=ORIENTED_EDGE('',*,*,#7844,.T.);
#10020=ORIENTED_EDGE('',*,*,#7845,.F.);
#10021=ORIENTED_EDGE('',*,*,#7840,.F.);
#10022=ORIENTED_EDGE('',*,*,#7846,.F.);
#10023=ORIENTED_EDGE('',*,*,#7847,.T.);
#10024=ORIENTED_EDGE('',*,*,#7848,.F.);
#10025=ORIENTED_EDGE('',*,*,#7844,.F.);
#10026=ORIENTED_EDGE('',*,*,#7849,.F.);
#10027=ORIENTED_EDGE('',*,*,#7850,.T.);
#10028=ORIENTED_EDGE('',*,*,#7851,.F.);
#10029=ORIENTED_EDGE('',*,*,#7847,.F.);
#10030=ORIENTED_EDGE('',*,*,#7852,.F.);
#10031=ORIENTED_EDGE('',*,*,#7853,.T.);
#10032=ORIENTED_EDGE('',*,*,#7854,.F.);
#10033=ORIENTED_EDGE('',*,*,#7850,.F.);
#10034=ORIENTED_EDGE('',*,*,#7855,.F.);
#10035=ORIENTED_EDGE('',*,*,#7856,.T.);
#10036=ORIENTED_EDGE('',*,*,#7857,.F.);
#10037=ORIENTED_EDGE('',*,*,#7853,.F.);
#10038=ORIENTED_EDGE('',*,*,#7858,.F.);
#10039=ORIENTED_EDGE('',*,*,#7859,.T.);
#10040=ORIENTED_EDGE('',*,*,#7860,.F.);
#10041=ORIENTED_EDGE('',*,*,#7856,.F.);
#10042=ORIENTED_EDGE('',*,*,#7861,.F.);
#10043=ORIENTED_EDGE('',*,*,#7862,.T.);
#10044=ORIENTED_EDGE('',*,*,#7863,.F.);
#10045=ORIENTED_EDGE('',*,*,#7859,.F.);
#10046=ORIENTED_EDGE('',*,*,#7864,.F.);
#10047=ORIENTED_EDGE('',*,*,#7865,.F.);
#10048=ORIENTED_EDGE('',*,*,#7866,.F.);
#10049=ORIENTED_EDGE('',*,*,#7862,.F.);
#10050=ORIENTED_EDGE('',*,*,#7867,.F.);
#10051=ORIENTED_EDGE('',*,*,#7868,.T.);
#10052=ORIENTED_EDGE('',*,*,#7869,.F.);
#10053=ORIENTED_EDGE('',*,*,#7870,.F.);
#10054=ORIENTED_EDGE('',*,*,#7871,.F.);
#10055=ORIENTED_EDGE('',*,*,#7872,.T.);
#10056=ORIENTED_EDGE('',*,*,#7873,.F.);
#10057=ORIENTED_EDGE('',*,*,#7868,.F.);
#10058=ORIENTED_EDGE('',*,*,#7874,.F.);
#10059=ORIENTED_EDGE('',*,*,#7875,.T.);
#10060=ORIENTED_EDGE('',*,*,#7876,.F.);
#10061=ORIENTED_EDGE('',*,*,#7872,.F.);
#10062=ORIENTED_EDGE('',*,*,#7877,.F.);
#10063=ORIENTED_EDGE('',*,*,#7878,.T.);
#10064=ORIENTED_EDGE('',*,*,#7879,.F.);
#10065=ORIENTED_EDGE('',*,*,#7875,.F.);
#10066=ORIENTED_EDGE('',*,*,#7880,.F.);
#10067=ORIENTED_EDGE('',*,*,#7881,.T.);
#10068=ORIENTED_EDGE('',*,*,#7882,.F.);
#10069=ORIENTED_EDGE('',*,*,#7878,.F.);
#10070=ORIENTED_EDGE('',*,*,#7883,.F.);
#10071=ORIENTED_EDGE('',*,*,#7884,.T.);
#10072=ORIENTED_EDGE('',*,*,#7885,.F.);
#10073=ORIENTED_EDGE('',*,*,#7881,.F.);
#10074=ORIENTED_EDGE('',*,*,#7886,.F.);
#10075=ORIENTED_EDGE('',*,*,#7887,.T.);
#10076=ORIENTED_EDGE('',*,*,#7888,.F.);
#10077=ORIENTED_EDGE('',*,*,#7884,.F.);
#10078=ORIENTED_EDGE('',*,*,#7889,.F.);
#10079=ORIENTED_EDGE('',*,*,#7890,.T.);
#10080=ORIENTED_EDGE('',*,*,#7891,.F.);
#10081=ORIENTED_EDGE('',*,*,#7887,.F.);
#10082=ORIENTED_EDGE('',*,*,#7892,.F.);
#10083=ORIENTED_EDGE('',*,*,#7893,.F.);
#10084=ORIENTED_EDGE('',*,*,#7894,.F.);
#10085=ORIENTED_EDGE('',*,*,#7890,.F.);
#10086=ORIENTED_EDGE('',*,*,#7895,.F.);
#10087=ORIENTED_EDGE('',*,*,#7896,.T.);
#10088=ORIENTED_EDGE('',*,*,#7897,.F.);
#10089=ORIENTED_EDGE('',*,*,#7896,.F.);
#10090=ORIENTED_EDGE('',*,*,#7809,.T.);
#10091=ORIENTED_EDGE('',*,*,#7898,.T.);
#10092=ORIENTED_EDGE('',*,*,#7899,.T.);
#10093=ORIENTED_EDGE('',*,*,#7900,.F.);
#10094=ORIENTED_EDGE('',*,*,#7786,.T.);
#10095=ORIENTED_EDGE('',*,*,#7901,.F.);
#10096=ORIENTED_EDGE('',*,*,#7902,.F.);
#10097=ORIENTED_EDGE('',*,*,#7903,.T.);
#10098=ORIENTED_EDGE('',*,*,#7837,.T.);
#10099=ORIENTED_EDGE('',*,*,#7904,.T.);
#10100=ORIENTED_EDGE('',*,*,#7902,.T.);
#10101=ORIENTED_EDGE('',*,*,#7905,.F.);
#10102=ORIENTED_EDGE('',*,*,#7814,.T.);
#10103=ORIENTED_EDGE('',*,*,#7906,.F.);
#10104=ORIENTED_EDGE('',*,*,#7907,.F.);
#10105=ORIENTED_EDGE('',*,*,#7908,.T.);
#10106=ORIENTED_EDGE('',*,*,#7865,.T.);
#10107=ORIENTED_EDGE('',*,*,#7909,.T.);
#10108=ORIENTED_EDGE('',*,*,#7907,.T.);
#10109=ORIENTED_EDGE('',*,*,#7910,.F.);
#10110=ORIENTED_EDGE('',*,*,#7842,.T.);
#10111=ORIENTED_EDGE('',*,*,#7911,.F.);
#10112=ORIENTED_EDGE('',*,*,#7912,.F.);
#10113=ORIENTED_EDGE('',*,*,#7913,.T.);
#10114=ORIENTED_EDGE('',*,*,#7893,.T.);
#10115=ORIENTED_EDGE('',*,*,#7914,.T.);
#10116=ORIENTED_EDGE('',*,*,#7912,.T.);
#10117=ORIENTED_EDGE('',*,*,#7915,.F.);
#10118=ORIENTED_EDGE('',*,*,#7870,.T.);
#10119=ORIENTED_EDGE('',*,*,#7916,.F.);
#10120=ORIENTED_EDGE('',*,*,#7899,.F.);
#10121=ORIENTED_EDGE('',*,*,#7917,.T.);
#10122=ORIENTED_EDGE('',*,*,#7785,.T.);
#10123=ORIENTED_EDGE('',*,*,#7789,.T.);
#10124=ORIENTED_EDGE('',*,*,#7792,.T.);
#10125=ORIENTED_EDGE('',*,*,#7795,.T.);
#10126=ORIENTED_EDGE('',*,*,#7798,.T.);
#10127=ORIENTED_EDGE('',*,*,#7801,.T.);
#10128=ORIENTED_EDGE('',*,*,#7804,.T.);
#10129=ORIENTED_EDGE('',*,*,#7807,.T.);
#10130=ORIENTED_EDGE('',*,*,#7810,.T.);
#10131=ORIENTED_EDGE('',*,*,#7900,.T.);
#10132=ORIENTED_EDGE('',*,*,#7916,.T.);
#10133=ORIENTED_EDGE('',*,*,#7869,.T.);
#10134=ORIENTED_EDGE('',*,*,#7873,.T.);
#10135=ORIENTED_EDGE('',*,*,#7876,.T.);
#10136=ORIENTED_EDGE('',*,*,#7879,.T.);
#10137=ORIENTED_EDGE('',*,*,#7882,.T.);
#10138=ORIENTED_EDGE('',*,*,#7885,.T.);
#10139=ORIENTED_EDGE('',*,*,#7888,.T.);
#10140=ORIENTED_EDGE('',*,*,#7891,.T.);
#10141=ORIENTED_EDGE('',*,*,#7894,.T.);
#10142=ORIENTED_EDGE('',*,*,#7915,.T.);
#10143=ORIENTED_EDGE('',*,*,#7911,.T.);
#10144=ORIENTED_EDGE('',*,*,#7841,.T.);
#10145=ORIENTED_EDGE('',*,*,#7845,.T.);
#10146=ORIENTED_EDGE('',*,*,#7848,.T.);
#10147=ORIENTED_EDGE('',*,*,#7851,.T.);
#10148=ORIENTED_EDGE('',*,*,#7854,.T.);
#10149=ORIENTED_EDGE('',*,*,#7857,.T.);
#10150=ORIENTED_EDGE('',*,*,#7860,.T.);
#10151=ORIENTED_EDGE('',*,*,#7863,.T.);
#10152=ORIENTED_EDGE('',*,*,#7866,.T.);
#10153=ORIENTED_EDGE('',*,*,#7910,.T.);
#10154=ORIENTED_EDGE('',*,*,#7906,.T.);
#10155=ORIENTED_EDGE('',*,*,#7813,.T.);
#10156=ORIENTED_EDGE('',*,*,#7817,.T.);
#10157=ORIENTED_EDGE('',*,*,#7820,.T.);
#10158=ORIENTED_EDGE('',*,*,#7823,.T.);
#10159=ORIENTED_EDGE('',*,*,#7826,.T.);
#10160=ORIENTED_EDGE('',*,*,#7829,.T.);
#10161=ORIENTED_EDGE('',*,*,#7832,.T.);
#10162=ORIENTED_EDGE('',*,*,#7835,.T.);
#10163=ORIENTED_EDGE('',*,*,#7838,.T.);
#10164=ORIENTED_EDGE('',*,*,#7905,.T.);
#10165=ORIENTED_EDGE('',*,*,#7901,.T.);
#10166=ORIENTED_EDGE('',*,*,#7897,.T.);
#10167=ORIENTED_EDGE('',*,*,#7783,.T.);
#10168=ORIENTED_EDGE('',*,*,#7903,.F.);
#10169=ORIENTED_EDGE('',*,*,#7904,.F.);
#10170=ORIENTED_EDGE('',*,*,#7836,.T.);
#10171=ORIENTED_EDGE('',*,*,#7833,.T.);
#10172=ORIENTED_EDGE('',*,*,#7830,.T.);
#10173=ORIENTED_EDGE('',*,*,#7827,.T.);
#10174=ORIENTED_EDGE('',*,*,#7824,.T.);
#10175=ORIENTED_EDGE('',*,*,#7821,.T.);
#10176=ORIENTED_EDGE('',*,*,#7818,.T.);
#10177=ORIENTED_EDGE('',*,*,#7815,.T.);
#10178=ORIENTED_EDGE('',*,*,#7811,.T.);
#10179=ORIENTED_EDGE('',*,*,#7908,.F.);
#10180=ORIENTED_EDGE('',*,*,#7909,.F.);
#10181=ORIENTED_EDGE('',*,*,#7864,.T.);
#10182=ORIENTED_EDGE('',*,*,#7861,.T.);
#10183=ORIENTED_EDGE('',*,*,#7858,.T.);
#10184=ORIENTED_EDGE('',*,*,#7855,.T.);
#10185=ORIENTED_EDGE('',*,*,#7852,.T.);
#10186=ORIENTED_EDGE('',*,*,#7849,.T.);
#10187=ORIENTED_EDGE('',*,*,#7846,.T.);
#10188=ORIENTED_EDGE('',*,*,#7843,.T.);
#10189=ORIENTED_EDGE('',*,*,#7839,.T.);
#10190=ORIENTED_EDGE('',*,*,#7913,.F.);
#10191=ORIENTED_EDGE('',*,*,#7914,.F.);
#10192=ORIENTED_EDGE('',*,*,#7892,.T.);
#10193=ORIENTED_EDGE('',*,*,#7889,.T.);
#10194=ORIENTED_EDGE('',*,*,#7886,.T.);
#10195=ORIENTED_EDGE('',*,*,#7883,.T.);
#10196=ORIENTED_EDGE('',*,*,#7880,.T.);
#10197=ORIENTED_EDGE('',*,*,#7877,.T.);
#10198=ORIENTED_EDGE('',*,*,#7874,.T.);
#10199=ORIENTED_EDGE('',*,*,#7871,.T.);
#10200=ORIENTED_EDGE('',*,*,#7867,.T.);
#10201=ORIENTED_EDGE('',*,*,#7917,.F.);
#10202=ORIENTED_EDGE('',*,*,#7898,.F.);
#10203=ORIENTED_EDGE('',*,*,#7808,.T.);
#10204=ORIENTED_EDGE('',*,*,#7805,.T.);
#10205=ORIENTED_EDGE('',*,*,#7802,.T.);
#10206=ORIENTED_EDGE('',*,*,#7799,.T.);
#10207=ORIENTED_EDGE('',*,*,#7796,.T.);
#10208=ORIENTED_EDGE('',*,*,#7793,.T.);
#10209=ORIENTED_EDGE('',*,*,#7790,.T.);
#10210=ORIENTED_EDGE('',*,*,#7787,.T.);
#10211=ORIENTED_EDGE('',*,*,#7895,.T.);
#12914=CYLINDRICAL_SURFACE('',#14664,0.21);
#13167=ADVANCED_FACE('',(#1689),#1128,.F.);
#13168=ADVANCED_FACE('',(#1690),#1129,.F.);
#13169=ADVANCED_FACE('',(#1691),#1130,.F.);
#13170=ADVANCED_FACE('',(#1692),#1131,.F.);
#13171=ADVANCED_FACE('',(#1693),#1132,.F.);
#13172=ADVANCED_FACE('',(#1694),#1133,.F.);
#13173=ADVANCED_FACE('',(#1695),#1134,.F.);
#13174=ADVANCED_FACE('',(#1696),#1135,.F.);
#13175=ADVANCED_FACE('',(#1697),#1136,.F.);
#13176=ADVANCED_FACE('',(#1698),#1137,.F.);
#13177=ADVANCED_FACE('',(#1699),#1138,.F.);
#13178=ADVANCED_FACE('',(#1700),#1139,.F.);
#13179=ADVANCED_FACE('',(#1701),#1140,.F.);
#13180=ADVANCED_FACE('',(#1702),#1141,.F.);
#13181=ADVANCED_FACE('',(#1703),#1142,.F.);
#13182=ADVANCED_FACE('',(#1704),#1143,.F.);
#13183=ADVANCED_FACE('',(#1705),#1144,.F.);
#13184=ADVANCED_FACE('',(#1706),#1145,.F.);
#13185=ADVANCED_FACE('',(#1707),#1146,.F.);
#13186=ADVANCED_FACE('',(#1708),#1147,.F.);
#13187=ADVANCED_FACE('',(#1709),#1148,.F.);
#13188=ADVANCED_FACE('',(#1710),#1149,.F.);
#13189=ADVANCED_FACE('',(#1711),#1150,.F.);
#13190=ADVANCED_FACE('',(#1712),#1151,.F.);
#13191=ADVANCED_FACE('',(#1713),#1152,.F.);
#13192=ADVANCED_FACE('',(#1714),#1153,.F.);
#13193=ADVANCED_FACE('',(#1715),#1154,.F.);
#13194=ADVANCED_FACE('',(#1716),#1155,.F.);
#13195=ADVANCED_FACE('',(#1717),#1156,.F.);
#13196=ADVANCED_FACE('',(#1718),#1157,.F.);
#13197=ADVANCED_FACE('',(#1719),#1158,.F.);
#13198=ADVANCED_FACE('',(#1720),#1159,.F.);
#13199=ADVANCED_FACE('',(#1721),#1160,.F.);
#13200=ADVANCED_FACE('',(#1722),#1161,.F.);
#13201=ADVANCED_FACE('',(#1723),#1162,.F.);
#13202=ADVANCED_FACE('',(#1724),#1163,.F.);
#13203=ADVANCED_FACE('',(#1725),#12914,.F.);
#13204=ADVANCED_FACE('',(#1726),#1164,.T.);
#13205=ADVANCED_FACE('',(#1727),#1165,.T.);
#13206=ADVANCED_FACE('',(#1728),#1166,.T.);
#13207=ADVANCED_FACE('',(#1729),#1167,.T.);
#13208=ADVANCED_FACE('',(#1730),#1168,.T.);
#13209=ADVANCED_FACE('',(#1731),#1169,.T.);
#13210=ADVANCED_FACE('',(#1732),#1170,.T.);
#13211=ADVANCED_FACE('',(#1733),#1171,.T.);
#13212=ADVANCED_FACE('',(#1734,#957),#1172,.T.);
#13213=ADVANCED_FACE('',(#1735,#958),#1173,.F.);
#13766=CLOSED_SHELL('',(#13167,#13168,#13169,#13170,#13171,#13172,#13173,
#13174,#13175,#13176,#13177,#13178,#13179,#13180,#13181,#13182,#13183,#13184,
#13185,#13186,#13187,#13188,#13189,#13190,#13191,#13192,#13193,#13194,#13195,
#13196,#13197,#13198,#13199,#13200,#13201,#13202,#13203,#13204,#13205,#13206,
#13207,#13208,#13209,#13210,#13211,#13212,#13213));
#14627=AXIS2_PLACEMENT_3D('',#20217,#16434,#16435);
#14628=AXIS2_PLACEMENT_3D('',#20218,#16436,#16437);
#14629=AXIS2_PLACEMENT_3D('',#20227,#16442,#16443);
#14630=AXIS2_PLACEMENT_3D('',#20233,#16447,#16448);
#14631=AXIS2_PLACEMENT_3D('',#20239,#16452,#16453);
#14632=AXIS2_PLACEMENT_3D('',#20245,#16457,#16458);
#14633=AXIS2_PLACEMENT_3D('',#20251,#16462,#16463);
#14634=AXIS2_PLACEMENT_3D('',#20257,#16467,#16468);
#14635=AXIS2_PLACEMENT_3D('',#20263,#16472,#16473);
#14636=AXIS2_PLACEMENT_3D('',#20269,#16477,#16478);
#14637=AXIS2_PLACEMENT_3D('',#20275,#16482,#16483);
#14638=AXIS2_PLACEMENT_3D('',#20284,#16488,#16489);
#14639=AXIS2_PLACEMENT_3D('',#20290,#16493,#16494);
#14640=AXIS2_PLACEMENT_3D('',#20296,#16498,#16499);
#14641=AXIS2_PLACEMENT_3D('',#20302,#16503,#16504);
#14642=AXIS2_PLACEMENT_3D('',#20308,#16508,#16509);
#14643=AXIS2_PLACEMENT_3D('',#20314,#16513,#16514);
#14644=AXIS2_PLACEMENT_3D('',#20320,#16518,#16519);
#14645=AXIS2_PLACEMENT_3D('',#20326,#16523,#16524);
#14646=AXIS2_PLACEMENT_3D('',#20332,#16528,#16529);
#14647=AXIS2_PLACEMENT_3D('',#20341,#16534,#16535);
#14648=AXIS2_PLACEMENT_3D('',#20347,#16539,#16540);
#14649=AXIS2_PLACEMENT_3D('',#20353,#16544,#16545);
#14650=AXIS2_PLACEMENT_3D('',#20359,#16549,#16550);
#14651=AXIS2_PLACEMENT_3D('',#20365,#16554,#16555);
#14652=AXIS2_PLACEMENT_3D('',#20371,#16559,#16560);
#14653=AXIS2_PLACEMENT_3D('',#20377,#16564,#16565);
#14654=AXIS2_PLACEMENT_3D('',#20383,#16569,#16570);
#14655=AXIS2_PLACEMENT_3D('',#20389,#16574,#16575);
#14656=AXIS2_PLACEMENT_3D('',#20398,#16580,#16581);
#14657=AXIS2_PLACEMENT_3D('',#20404,#16585,#16586);
#14658=AXIS2_PLACEMENT_3D('',#20410,#16590,#16591);
#14659=AXIS2_PLACEMENT_3D('',#20416,#16595,#16596);
#14660=AXIS2_PLACEMENT_3D('',#20422,#16600,#16601);
#14661=AXIS2_PLACEMENT_3D('',#20428,#16605,#16606);
#14662=AXIS2_PLACEMENT_3D('',#20434,#16610,#16611);
#14663=AXIS2_PLACEMENT_3D('',#20440,#16615,#16616);
#14664=AXIS2_PLACEMENT_3D('',#20446,#16620,#16621);
#14665=AXIS2_PLACEMENT_3D('',#20448,#16622,#16623);
#14666=AXIS2_PLACEMENT_3D('',#20451,#16625,#16626);
#14667=AXIS2_PLACEMENT_3D('',#20452,#16627,#16628);
#14668=AXIS2_PLACEMENT_3D('',#20458,#16632,#16633);
#14669=AXIS2_PLACEMENT_3D('',#20464,#16637,#16638);
#14670=AXIS2_PLACEMENT_3D('',#20467,#16641,#16642);
#14671=AXIS2_PLACEMENT_3D('',#20473,#16646,#16647);
#14672=AXIS2_PLACEMENT_3D('',#20476,#16650,#16651);
#14673=AXIS2_PLACEMENT_3D('',#20482,#16655,#16656);
#14674=AXIS2_PLACEMENT_3D('',#20485,#16659,#16660);
#14675=AXIS2_PLACEMENT_3D('',#20488,#16663,#16664);
#14676=AXIS2_PLACEMENT_3D('',#20489,#16665,#16666);
#16434=DIRECTION('axis',(0.,0.,1.));
#16435=DIRECTION('refdir',(1.,0.,0.));
#16436=DIRECTION('center_axis',(0.,0.,-1.));
#16437=DIRECTION('ref_axis',(0.,1.,0.));
#16438=DIRECTION('',(0.,1.,0.));
#16439=DIRECTION('',(1.,0.,0.));
#16440=DIRECTION('',(0.,-1.,0.));
#16441=DIRECTION('',(1.,0.,0.));
#16442=DIRECTION('center_axis',(0.,1.,-8.88178419700125E-16));
#16443=DIRECTION('ref_axis',(0.,8.88178419700125E-16,1.));
#16444=DIRECTION('',(0.,8.88178419700125E-16,1.));
#16445=DIRECTION('',(1.,0.,0.));
#16446=DIRECTION('',(0.,-8.88178419700125E-16,-1.));
#16447=DIRECTION('center_axis',(0.,-7.40148683083439E-16,-1.));
#16448=DIRECTION('ref_axis',(0.,1.,-7.40148683083439E-16));
#16449=DIRECTION('',(0.,1.,-7.40148683083439E-16));
#16450=DIRECTION('',(1.,0.,0.));
#16451=DIRECTION('',(0.,-1.,7.40148683083439E-16));
#16452=DIRECTION('center_axis',(0.,-0.707106781186547,-0.707106781186548));
#16453=DIRECTION('ref_axis',(0.,0.707106781186548,-0.707106781186547));
#16454=DIRECTION('',(0.,0.707106781186548,-0.707106781186547));
#16455=DIRECTION('',(1.,0.,0.));
#16456=DIRECTION('',(0.,-0.707106781186548,0.707106781186547));
#16457=DIRECTION('center_axis',(0.,-1.,2.77555756156289E-16));
#16458=DIRECTION('ref_axis',(0.,-2.77555756156289E-16,-1.));
#16459=DIRECTION('',(0.,-2.77555756156289E-16,-1.));
#16460=DIRECTION('',(1.,0.,0.));
#16461=DIRECTION('',(0.,2.77555756156289E-16,1.));
#16462=DIRECTION('center_axis',(0.,-0.707106781186547,0.707106781186548));
#16463=DIRECTION('ref_axis',(0.,-0.707106781186548,-0.707106781186547));
#16464=DIRECTION('',(0.,-0.707106781186548,-0.707106781186547));
#16465=DIRECTION('',(1.,0.,0.));
#16466=DIRECTION('',(0.,0.707106781186548,0.707106781186547));
#16467=DIRECTION('center_axis',(0.,7.40148683083438E-16,1.));
#16468=DIRECTION('ref_axis',(0.,-1.,7.40148683083438E-16));
#16469=DIRECTION('',(0.,-1.,7.40148683083438E-16));
#16470=DIRECTION('',(1.,0.,0.));
#16471=DIRECTION('',(0.,1.,-7.40148683083438E-16));
#16472=DIRECTION('center_axis',(0.,1.,-4.44089209850063E-16));
#16473=DIRECTION('ref_axis',(0.,4.44089209850063E-16,1.));
#16474=DIRECTION('',(0.,4.44089209850063E-16,1.));
#16475=DIRECTION('',(1.,0.,0.));
#16476=DIRECTION('',(0.,-4.44089209850063E-16,-1.));
#16477=DIRECTION('center_axis',(0.,2.41352831440251E-16,1.));
#16478=DIRECTION('ref_axis',(0.,-1.,2.41352831440251E-16));
#16479=DIRECTION('',(0.,-1.,2.41352831440251E-16));
#16480=DIRECTION('',(-1.,0.,0.));
#16481=DIRECTION('',(0.,1.,-2.41352831440251E-16));
#16482=DIRECTION('center_axis',(0.,-1.,2.41352831440251E-16));
#16483=DIRECTION('ref_axis',(0.,-2.41352831440251E-16,-1.));
#16484=DIRECTION('',(0.,-2.41352831440251E-16,-1.));
#16485=DIRECTION('',(1.,0.,0.));
#16486=DIRECTION('',(0.,2.41352831440251E-16,1.));
#16487=DIRECTION('',(1.,0.,0.));
#16488=DIRECTION('center_axis',(0.,0.,-1.));
#16489=DIRECTION('ref_axis',(0.,1.,0.));
#16490=DIRECTION('',(0.,1.,0.));
#16491=DIRECTION('',(1.,0.,0.));
#16492=DIRECTION('',(0.,-1.,0.));
#16493=DIRECTION('center_axis',(0.,-1.,0.));
#16494=DIRECTION('ref_axis',(0.,0.,-1.));
#16495=DIRECTION('',(0.,0.,-1.));
#16496=DIRECTION('',(1.,0.,0.));
#16497=DIRECTION('',(0.,0.,1.));
#16498=DIRECTION('center_axis',(0.,-0.707106781186547,0.707106781186548));
#16499=DIRECTION('ref_axis',(0.,-0.707106781186548,-0.707106781186547));
#16500=DIRECTION('',(0.,-0.707106781186548,-0.707106781186547));
#16501=DIRECTION('',(1.,0.,0.));
#16502=DIRECTION('',(0.,0.707106781186548,0.707106781186547));
#16503=DIRECTION('center_axis',(0.,0.,1.));
#16504=DIRECTION('ref_axis',(0.,-1.,0.));
#16505=DIRECTION('',(0.,-1.,0.));
#16506=DIRECTION('',(1.,0.,0.));
#16507=DIRECTION('',(0.,1.,0.));
#16508=DIRECTION('center_axis',(0.,0.707106781186548,0.707106781186547));
#16509=DIRECTION('ref_axis',(0.,-0.707106781186547,0.707106781186548));
#16510=DIRECTION('',(0.,-0.707106781186547,0.707106781186548));
#16511=DIRECTION('',(1.,0.,0.));
#16512=DIRECTION('',(0.,0.707106781186547,-0.707106781186548));
#16513=DIRECTION('center_axis',(0.,1.,0.));
#16514=DIRECTION('ref_axis',(0.,0.,1.));
#16515=DIRECTION('',(0.,0.,1.));
#16516=DIRECTION('',(1.,0.,0.));
#16517=DIRECTION('',(0.,0.,-1.));
#16518=DIRECTION('center_axis',(0.,0.,-1.));
#16519=DIRECTION('ref_axis',(0.,1.,0.));
#16520=DIRECTION('',(0.,1.,0.));
#16521=DIRECTION('',(1.,0.,0.));
#16522=DIRECTION('',(0.,-1.,0.));
#16523=DIRECTION('center_axis',(0.,1.,-2.41352831440251E-16));
#16524=DIRECTION('ref_axis',(0.,2.41352831440251E-16,1.));
#16525=DIRECTION('',(0.,2.41352831440251E-16,1.));
#16526=DIRECTION('',(-1.,0.,0.));
#16527=DIRECTION('',(0.,-2.41352831440251E-16,-1.));
#16528=DIRECTION('center_axis',(0.,0.,1.));
#16529=DIRECTION('ref_axis',(0.,-1.,0.));
#16530=DIRECTION('',(0.,-1.,0.));
#16531=DIRECTION('',(1.,0.,0.));
#16532=DIRECTION('',(0.,1.,0.));
#16533=DIRECTION('',(1.,0.,0.));
#16534=DIRECTION('center_axis',(0.,-1.,0.));
#16535=DIRECTION('ref_axis',(0.,0.,-1.));
#16536=DIRECTION('',(0.,0.,-1.));
#16537=DIRECTION('',(1.,0.,0.));
#16538=DIRECTION('',(0.,0.,1.));
#16539=DIRECTION('center_axis',(0.,0.,1.));
#16540=DIRECTION('ref_axis',(0.,-1.,0.));
#16541=DIRECTION('',(0.,-1.,0.));
#16542=DIRECTION('',(1.,0.,0.));
#16543=DIRECTION('',(0.,1.,0.));
#16544=DIRECTION('center_axis',(0.,0.707106781186548,0.707106781186548));
#16545=DIRECTION('ref_axis',(0.,-0.707106781186548,0.707106781186548));
#16546=DIRECTION('',(0.,-0.707106781186548,0.707106781186548));
#16547=DIRECTION('',(1.,0.,0.));
#16548=DIRECTION('',(0.,0.707106781186548,-0.707106781186548));
#16549=DIRECTION('center_axis',(0.,1.,0.));
#16550=DIRECTION('ref_axis',(0.,0.,1.));
#16551=DIRECTION('',(0.,0.,1.));
#16552=DIRECTION('',(1.,0.,0.));
#16553=DIRECTION('',(0.,0.,-1.));
#16554=DIRECTION('center_axis',(0.,0.707106781186548,-0.707106781186547));
#16555=DIRECTION('ref_axis',(0.,0.707106781186547,0.707106781186548));
#16556=DIRECTION('',(0.,0.707106781186547,0.707106781186548));
#16557=DIRECTION('',(1.,0.,0.));
#16558=DIRECTION('',(0.,-0.707106781186547,-0.707106781186548));
#16559=DIRECTION('center_axis',(0.,-7.40148683083438E-16,-1.));
#16560=DIRECTION('ref_axis',(0.,1.,-7.40148683083438E-16));
#16561=DIRECTION('',(0.,1.,-7.40148683083438E-16));
#16562=DIRECTION('',(1.,0.,0.));
#16563=DIRECTION('',(0.,-1.,7.40148683083438E-16));
#16564=DIRECTION('center_axis',(0.,-1.,0.));
#16565=DIRECTION('ref_axis',(0.,0.,-1.));
#16566=DIRECTION('',(0.,0.,-1.));
#16567=DIRECTION('',(1.,0.,0.));
#16568=DIRECTION('',(0.,0.,1.));
#16569=DIRECTION('center_axis',(0.,0.,-1.));
#16570=DIRECTION('ref_axis',(0.,1.,0.));
#16571=DIRECTION('',(0.,1.,0.));
#16572=DIRECTION('',(-1.,0.,0.));
#16573=DIRECTION('',(0.,-1.,0.));
#16574=DIRECTION('center_axis',(0.,1.,0.));
#16575=DIRECTION('ref_axis',(0.,0.,1.));
#16576=DIRECTION('',(0.,0.,1.));
#16577=DIRECTION('',(1.,0.,0.));
#16578=DIRECTION('',(0.,0.,-1.));
#16579=DIRECTION('',(1.,0.,0.));
#16580=DIRECTION('center_axis',(0.,0.,1.));
#16581=DIRECTION('ref_axis',(0.,-1.,0.));
#16582=DIRECTION('',(0.,-1.,0.));
#16583=DIRECTION('',(1.,0.,0.));
#16584=DIRECTION('',(0.,1.,0.));
#16585=DIRECTION('center_axis',(0.,1.,0.));
#16586=DIRECTION('ref_axis',(0.,0.,1.));
#16587=DIRECTION('',(0.,0.,1.));
#16588=DIRECTION('',(1.,0.,0.));
#16589=DIRECTION('',(0.,0.,-1.));
#16590=DIRECTION('center_axis',(0.,0.707106781186547,-0.707106781186548));
#16591=DIRECTION('ref_axis',(0.,0.707106781186548,0.707106781186547));
#16592=DIRECTION('',(0.,0.707106781186548,0.707106781186547));
#16593=DIRECTION('',(1.,0.,0.));
#16594=DIRECTION('',(0.,-0.707106781186548,-0.707106781186547));
#16595=DIRECTION('center_axis',(0.,0.,-1.));
#16596=DIRECTION('ref_axis',(0.,1.,0.));
#16597=DIRECTION('',(0.,1.,0.));
#16598=DIRECTION('',(1.,0.,0.));
#16599=DIRECTION('',(0.,-1.,0.));
#16600=DIRECTION('center_axis',(0.,-0.707106781186547,-0.707106781186548));
#16601=DIRECTION('ref_axis',(0.,0.707106781186548,-0.707106781186547));
#16602=DIRECTION('',(0.,0.707106781186548,-0.707106781186547));
#16603=DIRECTION('',(1.,0.,0.));
#16604=DIRECTION('',(0.,-0.707106781186548,0.707106781186547));
#16605=DIRECTION('center_axis',(0.,-1.,0.));
#16606=DIRECTION('ref_axis',(0.,0.,-1.));
#16607=DIRECTION('',(0.,0.,-1.));
#16608=DIRECTION('',(1.,0.,0.));
#16609=DIRECTION('',(0.,0.,1.));
#16610=DIRECTION('center_axis',(0.,0.,1.));
#16611=DIRECTION('ref_axis',(0.,-1.,0.));
#16612=DIRECTION('',(0.,-1.,0.));
#16613=DIRECTION('',(1.,0.,0.));
#16614=DIRECTION('',(0.,1.,0.));
#16615=DIRECTION('center_axis',(0.,-1.,0.));
#16616=DIRECTION('ref_axis',(0.,0.,-1.));
#16617=DIRECTION('',(0.,0.,-1.));
#16618=DIRECTION('',(-1.,0.,0.));
#16619=DIRECTION('',(0.,0.,1.));
#16620=DIRECTION('center_axis',(1.,0.,0.));
#16621=DIRECTION('ref_axis',(0.,0.,-1.));
#16622=DIRECTION('center_axis',(1.,0.,0.));
#16623=DIRECTION('ref_axis',(0.,0.,-1.));
#16624=DIRECTION('',(1.,0.,0.));
#16625=DIRECTION('center_axis',(-1.,0.,0.));
#16626=DIRECTION('ref_axis',(0.,0.,-1.));
#16627=DIRECTION('center_axis',(0.,1.,0.));
#16628=DIRECTION('ref_axis',(0.,0.,1.));
#16629=DIRECTION('',(0.,0.,1.));
#16630=DIRECTION('',(1.,0.,0.));
#16631=DIRECTION('',(0.,0.,1.));
#16632=DIRECTION('center_axis',(0.,1.,0.));
#16633=DIRECTION('ref_axis',(0.,0.,1.));
#16634=DIRECTION('',(0.,0.,1.));
#16635=DIRECTION('',(1.,0.,0.));
#16636=DIRECTION('',(0.,0.,1.));
#16637=DIRECTION('center_axis',(0.,0.,-1.));
#16638=DIRECTION('ref_axis',(0.,1.,0.));
#16639=DIRECTION('',(0.,1.,0.));
#16640=DIRECTION('',(0.,1.,0.));
#16641=DIRECTION('center_axis',(0.,0.,-1.));
#16642=DIRECTION('ref_axis',(0.,1.,0.));
#16643=DIRECTION('',(0.,1.,0.));
#16644=DIRECTION('',(1.,0.,0.));
#16645=DIRECTION('',(0.,1.,0.));
#16646=DIRECTION('center_axis',(0.,-1.,0.));
#16647=DIRECTION('ref_axis',(0.,0.,-1.));
#16648=DIRECTION('',(0.,0.,-1.));
#16649=DIRECTION('',(0.,0.,-1.));
#16650=DIRECTION('center_axis',(0.,-1.,0.));
#16651=DIRECTION('ref_axis',(0.,0.,-1.));
#16652=DIRECTION('',(0.,0.,-1.));
#16653=DIRECTION('',(1.,0.,0.));
#16654=DIRECTION('',(0.,0.,-1.));
#16655=DIRECTION('center_axis',(0.,0.,1.));
#16656=DIRECTION('ref_axis',(0.,-1.,0.));
#16657=DIRECTION('',(0.,-1.,0.));
#16658=DIRECTION('',(0.,-1.,0.));
#16659=DIRECTION('center_axis',(0.,0.,1.));
#16660=DIRECTION('ref_axis',(0.,-1.,0.));
#16661=DIRECTION('',(0.,-1.,0.));
#16662=DIRECTION('',(0.,-1.,0.));
#16663=DIRECTION('center_axis',(1.,0.,0.));
#16664=DIRECTION('ref_axis',(0.,0.,-1.));
#16665=DIRECTION('center_axis',(1.,0.,0.));
#16666=DIRECTION('ref_axis',(0.,0.,-1.));
#20217=CARTESIAN_POINT('',(0.,0.,0.));
#20218=CARTESIAN_POINT('Origin',(-0.1,0.82,-0.3));
#20219=CARTESIAN_POINT('',(0.,0.82,-0.3));
#20220=CARTESIAN_POINT('',(0.,1.,-0.3));
#20221=CARTESIAN_POINT('',(0.,0.41,-0.3));
#20222=CARTESIAN_POINT('',(20.,0.82,-0.3));
#20223=CARTESIAN_POINT('',(-0.1,0.82,-0.3));
#20224=CARTESIAN_POINT('',(20.,1.,-0.3));
#20225=CARTESIAN_POINT('',(20.,0.41,-0.3));
#20226=CARTESIAN_POINT('',(-0.05,1.,-0.3));
#20227=CARTESIAN_POINT('Origin',(-0.1,0.82,-0.55));
#20228=CARTESIAN_POINT('',(0.,0.82,-0.55));
#20229=CARTESIAN_POINT('',(0.,0.82,-0.275));
#20230=CARTESIAN_POINT('',(20.,0.82,-0.55));
#20231=CARTESIAN_POINT('',(-0.1,0.82,-0.55));
#20232=CARTESIAN_POINT('',(20.,0.82,-0.275));
#20233=CARTESIAN_POINT('Origin',(-0.1,0.67,-0.55));
#20234=CARTESIAN_POINT('',(0.,0.67,-0.55));
#20235=CARTESIAN_POINT('',(0.,0.335,-0.55));
#20236=CARTESIAN_POINT('',(20.,0.67,-0.55));
#20237=CARTESIAN_POINT('',(-0.1,0.67,-0.55));
#20238=CARTESIAN_POINT('',(20.,0.335,-0.55));
#20239=CARTESIAN_POINT('Origin',(-0.1,0.42,-0.3));
#20240=CARTESIAN_POINT('',(0.,0.42,-0.3));
#20241=CARTESIAN_POINT('',(0.,0.24,-0.12));
#20242=CARTESIAN_POINT('',(20.,0.42,-0.3));
#20243=CARTESIAN_POINT('',(-0.1,0.42,-0.3));
#20244=CARTESIAN_POINT('',(20.,0.24,-0.12));
#20245=CARTESIAN_POINT('Origin',(-0.1,0.42,0.3));
#20246=CARTESIAN_POINT('',(0.,0.42,0.3));
#20247=CARTESIAN_POINT('',(0.,0.42,0.15));
#20248=CARTESIAN_POINT('',(20.,0.42,0.3));
#20249=CARTESIAN_POINT('',(-0.1,0.42,0.3));
#20250=CARTESIAN_POINT('',(20.,0.42,0.15));
#20251=CARTESIAN_POINT('Origin',(-0.1,0.67,0.55));
#20252=CARTESIAN_POINT('',(0.,0.67,0.55));
#20253=CARTESIAN_POINT('',(6.93889390390723E-18,0.365,0.245));
#20254=CARTESIAN_POINT('',(20.,0.67,0.55));
#20255=CARTESIAN_POINT('',(-0.1,0.67,0.55));
#20256=CARTESIAN_POINT('',(20.,0.365,0.245));
#20257=CARTESIAN_POINT('Origin',(-0.1,0.82,0.55));
#20258=CARTESIAN_POINT('',(0.,0.82,0.55));
#20259=CARTESIAN_POINT('',(0.,0.41,0.55));
#20260=CARTESIAN_POINT('',(20.,0.82,0.55));
#20261=CARTESIAN_POINT('',(-0.1,0.82,0.55));
#20262=CARTESIAN_POINT('',(20.,0.41,0.55));
#20263=CARTESIAN_POINT('Origin',(-0.1,0.82,0.3));
#20264=CARTESIAN_POINT('',(0.,0.82,0.3));
#20265=CARTESIAN_POINT('',(0.,0.82,0.15));
#20266=CARTESIAN_POINT('',(20.,0.82,0.3));
#20267=CARTESIAN_POINT('',(-0.1,0.82,0.3));
#20268=CARTESIAN_POINT('',(20.,0.82,0.15));
#20269=CARTESIAN_POINT('Origin',(-0.1,1.05,0.3));
#20270=CARTESIAN_POINT('',(0.,1.,0.3));
#20271=CARTESIAN_POINT('',(0.,0.525,0.3));
#20272=CARTESIAN_POINT('',(20.,1.,0.3));
#20273=CARTESIAN_POINT('',(-0.05,1.,0.3));
#20274=CARTESIAN_POINT('',(20.,0.525,0.3));
#20275=CARTESIAN_POINT('Origin',(-0.1,-0.3,-0.82));
#20276=CARTESIAN_POINT('',(0.,-0.3,-0.82));
#20277=CARTESIAN_POINT('',(0.,-0.3,-1.));
#20278=CARTESIAN_POINT('',(0.,-0.3,-0.41));
#20279=CARTESIAN_POINT('',(20.,-0.3,-0.82));
#20280=CARTESIAN_POINT('',(-0.1,-0.3,-0.82));
#20281=CARTESIAN_POINT('',(20.,-0.3,-1.));
#20282=CARTESIAN_POINT('',(20.,-0.3,-0.41));
#20283=CARTESIAN_POINT('',(-0.05,-0.3,-1.));
#20284=CARTESIAN_POINT('Origin',(-0.1,-0.55,-0.82));
#20285=CARTESIAN_POINT('',(0.,-0.55,-0.82));
#20286=CARTESIAN_POINT('',(0.,-0.275,-0.82));
#20287=CARTESIAN_POINT('',(20.,-0.55,-0.82));
#20288=CARTESIAN_POINT('',(-0.1,-0.55,-0.82));
#20289=CARTESIAN_POINT('',(20.,-0.275,-0.82));
#20290=CARTESIAN_POINT('Origin',(-0.1,-0.55,-0.67));
#20291=CARTESIAN_POINT('',(0.,-0.55,-0.67));
#20292=CARTESIAN_POINT('',(0.,-0.55,-0.335));
#20293=CARTESIAN_POINT('',(20.,-0.55,-0.67));
#20294=CARTESIAN_POINT('',(-0.1,-0.55,-0.67));
#20295=CARTESIAN_POINT('',(20.,-0.55,-0.335));
#20296=CARTESIAN_POINT('Origin',(-0.1,-0.3,-0.42));
#20297=CARTESIAN_POINT('',(0.,-0.3,-0.42));
#20298=CARTESIAN_POINT('',(0.,-0.12,-0.24));
#20299=CARTESIAN_POINT('',(20.,-0.3,-0.42));
#20300=CARTESIAN_POINT('',(-0.1,-0.3,-0.42));
#20301=CARTESIAN_POINT('',(20.,-0.12,-0.24));
#20302=CARTESIAN_POINT('Origin',(-0.1,0.3,-0.42));
#20303=CARTESIAN_POINT('',(0.,0.3,-0.42));
#20304=CARTESIAN_POINT('',(0.,0.15,-0.42));
#20305=CARTESIAN_POINT('',(20.,0.3,-0.42));
#20306=CARTESIAN_POINT('',(-0.1,0.3,-0.42));
#20307=CARTESIAN_POINT('',(20.,0.15,-0.42));
#20308=CARTESIAN_POINT('Origin',(-0.1,0.55,-0.67));
#20309=CARTESIAN_POINT('',(0.,0.55,-0.67));
#20310=CARTESIAN_POINT('',(0.,0.245,-0.365));
#20311=CARTESIAN_POINT('',(20.,0.55,-0.67));
#20312=CARTESIAN_POINT('',(-0.1,0.55,-0.67));
#20313=CARTESIAN_POINT('',(20.,0.245,-0.365));
#20314=CARTESIAN_POINT('Origin',(-0.1,0.55,-0.82));
#20315=CARTESIAN_POINT('',(0.,0.55,-0.82));
#20316=CARTESIAN_POINT('',(0.,0.55,-0.41));
#20317=CARTESIAN_POINT('',(20.,0.55,-0.82));
#20318=CARTESIAN_POINT('',(-0.1,0.55,-0.82));
#20319=CARTESIAN_POINT('',(20.,0.55,-0.41));
#20320=CARTESIAN_POINT('Origin',(-0.1,0.3,-0.82));
#20321=CARTESIAN_POINT('',(0.,0.3,-0.82));
#20322=CARTESIAN_POINT('',(0.,0.15,-0.82));
#20323=CARTESIAN_POINT('',(20.,0.3,-0.82));
#20324=CARTESIAN_POINT('',(-0.1,0.3,-0.82));
#20325=CARTESIAN_POINT('',(20.,0.15,-0.82));
#20326=CARTESIAN_POINT('Origin',(-0.1,0.3,-1.05));
#20327=CARTESIAN_POINT('',(0.,0.3,-1.));
#20328=CARTESIAN_POINT('',(0.,0.3,-0.525));
#20329=CARTESIAN_POINT('',(20.,0.3,-1.));
#20330=CARTESIAN_POINT('',(-0.05,0.3,-1.));
#20331=CARTESIAN_POINT('',(20.,0.3,-0.525));
#20332=CARTESIAN_POINT('Origin',(-0.1,-0.82,0.3));
#20333=CARTESIAN_POINT('',(0.,-0.82,0.3));
#20334=CARTESIAN_POINT('',(0.,-1.,0.3));
#20335=CARTESIAN_POINT('',(0.,-0.41,0.3));
#20336=CARTESIAN_POINT('',(20.,-0.82,0.3));
#20337=CARTESIAN_POINT('',(-0.1,-0.82,0.3));
#20338=CARTESIAN_POINT('',(20.,-1.,0.3));
#20339=CARTESIAN_POINT('',(20.,-0.41,0.3));
#20340=CARTESIAN_POINT('',(-0.05,-1.,0.3));
#20341=CARTESIAN_POINT('Origin',(-0.1,-0.82,0.55));
#20342=CARTESIAN_POINT('',(0.,-0.82,0.55));
#20343=CARTESIAN_POINT('',(0.,-0.82,0.275));
#20344=CARTESIAN_POINT('',(20.,-0.82,0.55));
#20345=CARTESIAN_POINT('',(-0.1,-0.82,0.55));
#20346=CARTESIAN_POINT('',(20.,-0.82,0.275));
#20347=CARTESIAN_POINT('Origin',(-0.1,-0.67,0.55));
#20348=CARTESIAN_POINT('',(0.,-0.67,0.55));
#20349=CARTESIAN_POINT('',(0.,-0.335,0.55));
#20350=CARTESIAN_POINT('',(20.,-0.67,0.55));
#20351=CARTESIAN_POINT('',(-0.1,-0.67,0.55));
#20352=CARTESIAN_POINT('',(20.,-0.335,0.55));
#20353=CARTESIAN_POINT('Origin',(-0.1,-0.42,0.3));
#20354=CARTESIAN_POINT('',(0.,-0.42,0.3));
#20355=CARTESIAN_POINT('',(-6.93889390390723E-18,-0.24,0.12));
#20356=CARTESIAN_POINT('',(20.,-0.42,0.3));
#20357=CARTESIAN_POINT('',(-0.1,-0.42,0.3));
#20358=CARTESIAN_POINT('',(20.,-0.24,0.12));
#20359=CARTESIAN_POINT('Origin',(-0.1,-0.42,-0.3));
#20360=CARTESIAN_POINT('',(0.,-0.42,-0.3));
#20361=CARTESIAN_POINT('',(0.,-0.42,-0.15));
#20362=CARTESIAN_POINT('',(20.,-0.42,-0.3));
#20363=CARTESIAN_POINT('',(-0.1,-0.42,-0.3));
#20364=CARTESIAN_POINT('',(20.,-0.42,-0.15));
#20365=CARTESIAN_POINT('Origin',(-0.1,-0.67,-0.55));
#20366=CARTESIAN_POINT('',(0.,-0.67,-0.55));
#20367=CARTESIAN_POINT('',(0.,-0.365,-0.245));
#20368=CARTESIAN_POINT('',(20.,-0.67,-0.55));
#20369=CARTESIAN_POINT('',(-0.1,-0.67,-0.55));
#20370=CARTESIAN_POINT('',(20.,-0.365,-0.245));
#20371=CARTESIAN_POINT('Origin',(-0.1,-0.82,-0.55));
#20372=CARTESIAN_POINT('',(0.,-0.82,-0.55));
#20373=CARTESIAN_POINT('',(0.,-0.41,-0.55));
#20374=CARTESIAN_POINT('',(20.,-0.82,-0.55));
#20375=CARTESIAN_POINT('',(-0.1,-0.82,-0.55));
#20376=CARTESIAN_POINT('',(20.,-0.41,-0.55));
#20377=CARTESIAN_POINT('Origin',(-0.1,-0.82,-0.3));
#20378=CARTESIAN_POINT('',(0.,-0.82,-0.3));
#20379=CARTESIAN_POINT('',(0.,-0.82,-0.15));
#20380=CARTESIAN_POINT('',(20.,-0.82,-0.3));
#20381=CARTESIAN_POINT('',(-0.1,-0.82,-0.3));
#20382=CARTESIAN_POINT('',(20.,-0.82,-0.15));
#20383=CARTESIAN_POINT('Origin',(-0.1,-1.05,-0.3));
#20384=CARTESIAN_POINT('',(0.,-1.,-0.3));
#20385=CARTESIAN_POINT('',(0.,-0.525,-0.3));
#20386=CARTESIAN_POINT('',(20.,-1.,-0.3));
#20387=CARTESIAN_POINT('',(-0.05,-1.,-0.3));
#20388=CARTESIAN_POINT('',(20.,-0.525,-0.3));
#20389=CARTESIAN_POINT('Origin',(-0.1,0.3,0.82));
#20390=CARTESIAN_POINT('',(0.,0.3,0.82));
#20391=CARTESIAN_POINT('',(0.,0.3,1.));
#20392=CARTESIAN_POINT('',(0.,0.3,0.41));
#20393=CARTESIAN_POINT('',(20.,0.3,0.82));
#20394=CARTESIAN_POINT('',(-0.1,0.3,0.82));
#20395=CARTESIAN_POINT('',(20.,0.3,1.));
#20396=CARTESIAN_POINT('',(20.,0.3,0.41));
#20397=CARTESIAN_POINT('',(-0.05,0.3,1.));
#20398=CARTESIAN_POINT('Origin',(-0.1,0.55,0.82));
#20399=CARTESIAN_POINT('',(0.,0.55,0.82));
#20400=CARTESIAN_POINT('',(0.,0.275,0.82));
#20401=CARTESIAN_POINT('',(20.,0.55,0.82));
#20402=CARTESIAN_POINT('',(-0.1,0.55,0.82));
#20403=CARTESIAN_POINT('',(20.,0.275,0.82));
#20404=CARTESIAN_POINT('Origin',(-0.1,0.55,0.67));
#20405=CARTESIAN_POINT('',(0.,0.55,0.67));
#20406=CARTESIAN_POINT('',(0.,0.55,0.335));
#20407=CARTESIAN_POINT('',(20.,0.55,0.67));
#20408=CARTESIAN_POINT('',(-0.1,0.55,0.67));
#20409=CARTESIAN_POINT('',(20.,0.55,0.335));
#20410=CARTESIAN_POINT('Origin',(-0.1,0.3,0.42));
#20411=CARTESIAN_POINT('',(0.,0.3,0.42));
#20412=CARTESIAN_POINT('',(6.93889390390723E-18,0.12,0.24));
#20413=CARTESIAN_POINT('',(20.,0.3,0.42));
#20414=CARTESIAN_POINT('',(-0.1,0.3,0.42));
#20415=CARTESIAN_POINT('',(20.,0.12,0.24));
#20416=CARTESIAN_POINT('Origin',(-0.1,-0.3,0.42));
#20417=CARTESIAN_POINT('',(0.,-0.3,0.42));
#20418=CARTESIAN_POINT('',(0.,-0.15,0.42));
#20419=CARTESIAN_POINT('',(20.,-0.3,0.42));
#20420=CARTESIAN_POINT('',(-0.1,-0.3,0.42));
#20421=CARTESIAN_POINT('',(20.,-0.15,0.42));
#20422=CARTESIAN_POINT('Origin',(-0.1,-0.55,0.67));
#20423=CARTESIAN_POINT('',(0.,-0.55,0.67));
#20424=CARTESIAN_POINT('',(6.93889390390723E-18,-0.245,0.365));
#20425=CARTESIAN_POINT('',(20.,-0.55,0.67));
#20426=CARTESIAN_POINT('',(-0.1,-0.55,0.67));
#20427=CARTESIAN_POINT('',(20.,-0.245,0.365));
#20428=CARTESIAN_POINT('Origin',(-0.1,-0.55,0.82));
#20429=CARTESIAN_POINT('',(0.,-0.55,0.82));
#20430=CARTESIAN_POINT('',(0.,-0.55,0.41));
#20431=CARTESIAN_POINT('',(20.,-0.55,0.82));
#20432=CARTESIAN_POINT('',(-0.1,-0.55,0.82));
#20433=CARTESIAN_POINT('',(20.,-0.55,0.41));
#20434=CARTESIAN_POINT('Origin',(-0.1,-0.3,0.82));
#20435=CARTESIAN_POINT('',(0.,-0.3,0.82));
#20436=CARTESIAN_POINT('',(0.,-0.15,0.82));
#20437=CARTESIAN_POINT('',(20.,-0.3,0.82));
#20438=CARTESIAN_POINT('',(-0.1,-0.3,0.82));
#20439=CARTESIAN_POINT('',(20.,-0.15,0.82));
#20440=CARTESIAN_POINT('Origin',(-0.1,-0.3,1.05));
#20441=CARTESIAN_POINT('',(0.,-0.3,1.));
#20442=CARTESIAN_POINT('',(0.,-0.3,0.525));
#20443=CARTESIAN_POINT('',(20.,-0.3,1.));
#20444=CARTESIAN_POINT('',(-0.05,-0.3,1.));
#20445=CARTESIAN_POINT('',(20.,-0.3,0.525));
#20446=CARTESIAN_POINT('Origin',(-0.1,0.,0.));
#20447=CARTESIAN_POINT('',(0.,-2.57175827820944E-17,0.21));
#20448=CARTESIAN_POINT('Origin',(0.,0.,0.));
#20449=CARTESIAN_POINT('',(20.,2.57175827820944E-17,0.21));
#20450=CARTESIAN_POINT('',(-0.1,-2.57175827820944E-17,0.21));
#20451=CARTESIAN_POINT('Origin',(20.,0.,0.));
#20452=CARTESIAN_POINT('Origin',(0.,1.,-1.));
#20453=CARTESIAN_POINT('',(0.,1.,1.));
#20454=CARTESIAN_POINT('',(0.,1.,-1.));
#20455=CARTESIAN_POINT('',(20.,1.,1.));
#20456=CARTESIAN_POINT('',(0.,1.,1.));
#20457=CARTESIAN_POINT('',(20.,1.,-1.));
#20458=CARTESIAN_POINT('Origin',(0.,1.,-1.));
#20459=CARTESIAN_POINT('',(20.,1.,-1.));
#20460=CARTESIAN_POINT('',(20.,1.,-1.));
#20461=CARTESIAN_POINT('',(0.,1.,-1.));
#20462=CARTESIAN_POINT('',(0.,1.,-1.));
#20463=CARTESIAN_POINT('',(0.,1.,-1.));
#20464=CARTESIAN_POINT('Origin',(0.,-1.,-1.));
#20465=CARTESIAN_POINT('',(0.,-1.,-1.));
#20466=CARTESIAN_POINT('',(20.,-1.,-1.));
#20467=CARTESIAN_POINT('Origin',(0.,-1.,-1.));
#20468=CARTESIAN_POINT('',(20.,-1.,-1.));
#20469=CARTESIAN_POINT('',(20.,-1.,-1.));
#20470=CARTESIAN_POINT('',(0.,-1.,-1.));
#20471=CARTESIAN_POINT('',(0.,-1.,-1.));
#20472=CARTESIAN_POINT('',(0.,-1.,-1.));
#20473=CARTESIAN_POINT('Origin',(0.,-1.,1.));
#20474=CARTESIAN_POINT('',(0.,-1.,1.));
#20475=CARTESIAN_POINT('',(20.,-1.,1.));
#20476=CARTESIAN_POINT('Origin',(0.,-1.,1.));
#20477=CARTESIAN_POINT('',(20.,-1.,1.));
#20478=CARTESIAN_POINT('',(20.,-1.,1.));
#20479=CARTESIAN_POINT('',(0.,-1.,1.));
#20480=CARTESIAN_POINT('',(0.,-1.,1.));
#20481=CARTESIAN_POINT('',(0.,-1.,1.));
#20482=CARTESIAN_POINT('Origin',(0.,1.,1.));
#20483=CARTESIAN_POINT('',(0.,1.,1.));
#20484=CARTESIAN_POINT('',(20.,1.,1.));
#20485=CARTESIAN_POINT('Origin',(0.,1.,1.));
#20486=CARTESIAN_POINT('',(20.,1.,1.));
#20487=CARTESIAN_POINT('',(0.,1.,1.));
#20488=CARTESIAN_POINT('Origin',(20.,0.,0.));
#20489=CARTESIAN_POINT('Origin',(0.,0.,0.));
#34760=UNCERTAINTY_MEASURE_WITH_UNIT(LENGTH_MEASURE(0.001),#34852,
'DISTANCE_ACCURACY_VALUE',
'Maximum model space distance between geometric entities at asserted c
onnectivities');
#34797=UNCERTAINTY_MEASURE_WITH_UNIT(LENGTH_MEASURE(0.001),#34852,
'DISTANCE_ACCURACY_VALUE',
'Maximum model space distance between geometric entities at asserted c
onnectivities');
#34814=(
GEOMETRIC_REPRESENTATION_CONTEXT(3)
GLOBAL_UNCERTAINTY_ASSIGNED_CONTEXT((#34760))
GLOBAL_UNIT_ASSIGNED_CONTEXT((#34852,#34854,#34855))
REPRESENTATION_CONTEXT('','3D')
);
#34851=(
GEOMETRIC_REPRESENTATION_CONTEXT(3)
GLOBAL_UNCERTAINTY_ASSIGNED_CONTEXT((#34797))
GLOBAL_UNIT_ASSIGNED_CONTEXT((#34852,#34854,#34855))
REPRESENTATION_CONTEXT('','3D')
);
#34852=(
LENGTH_UNIT()
NAMED_UNIT(*)
SI_UNIT(.CENTI.,.METRE.)
);
#34854=(
NAMED_UNIT(*)
PLANE_ANGLE_UNIT()
SI_UNIT($,.RADIAN.)
);
#34855=(
NAMED_UNIT(*)
SI_UNIT($,.STERADIAN.)
SOLID_ANGLE_UNIT()
);
#34872=SHAPE_DEFINITION_REPRESENTATION(#34925,#35089);
#34925=PRODUCT_DEFINITION_SHAPE('',$,#35143);
#35089=SHAPE_REPRESENTATION('',(#14627),#34814);
#35126=PRODUCT_DEFINITION_CONTEXT('part definition',#35287,'design');
#35143=PRODUCT_DEFINITION('Slotted Extrusion - 20 x 20 x 200 mm',
'Slotted Extrusion - 20 x 20 x 200 mm',#35196,#35126);
#35196=PRODUCT_DEFINITION_FORMATION('',$,#35305);
#35287=APPLICATION_CONTEXT(
'Core Data for Automotive Mechanical Design Process');
#35288=PRODUCT_CONTEXT('part definition',#35287,'mechanical');
#35305=PRODUCT('Slotted Extrusion - 20 x 20 x 200 mm',
'Slotted Extrusion - 20 x 20 x 200 mm',
'Slotted Extrusion - 20 x 20 x 200 mm',(#35288));
#35419=COLOUR_RGB('Off White',0.89,0.88,0.83);
#35420=FILL_AREA_STYLE_COLOUR('',#35419);
#35421=FILL_AREA_STYLE('',(#35420));
#35422=SURFACE_STYLE_FILL_AREA(#35421);
#35423=SURFACE_SIDE_STYLE('',(#35422));
#35424=SURFACE_STYLE_USAGE(.BOTH.,#35423);
#35425=PRESENTATION_STYLE_ASSIGNMENT((#35424));
ENDSEC;
END-ISO-10303-21;
